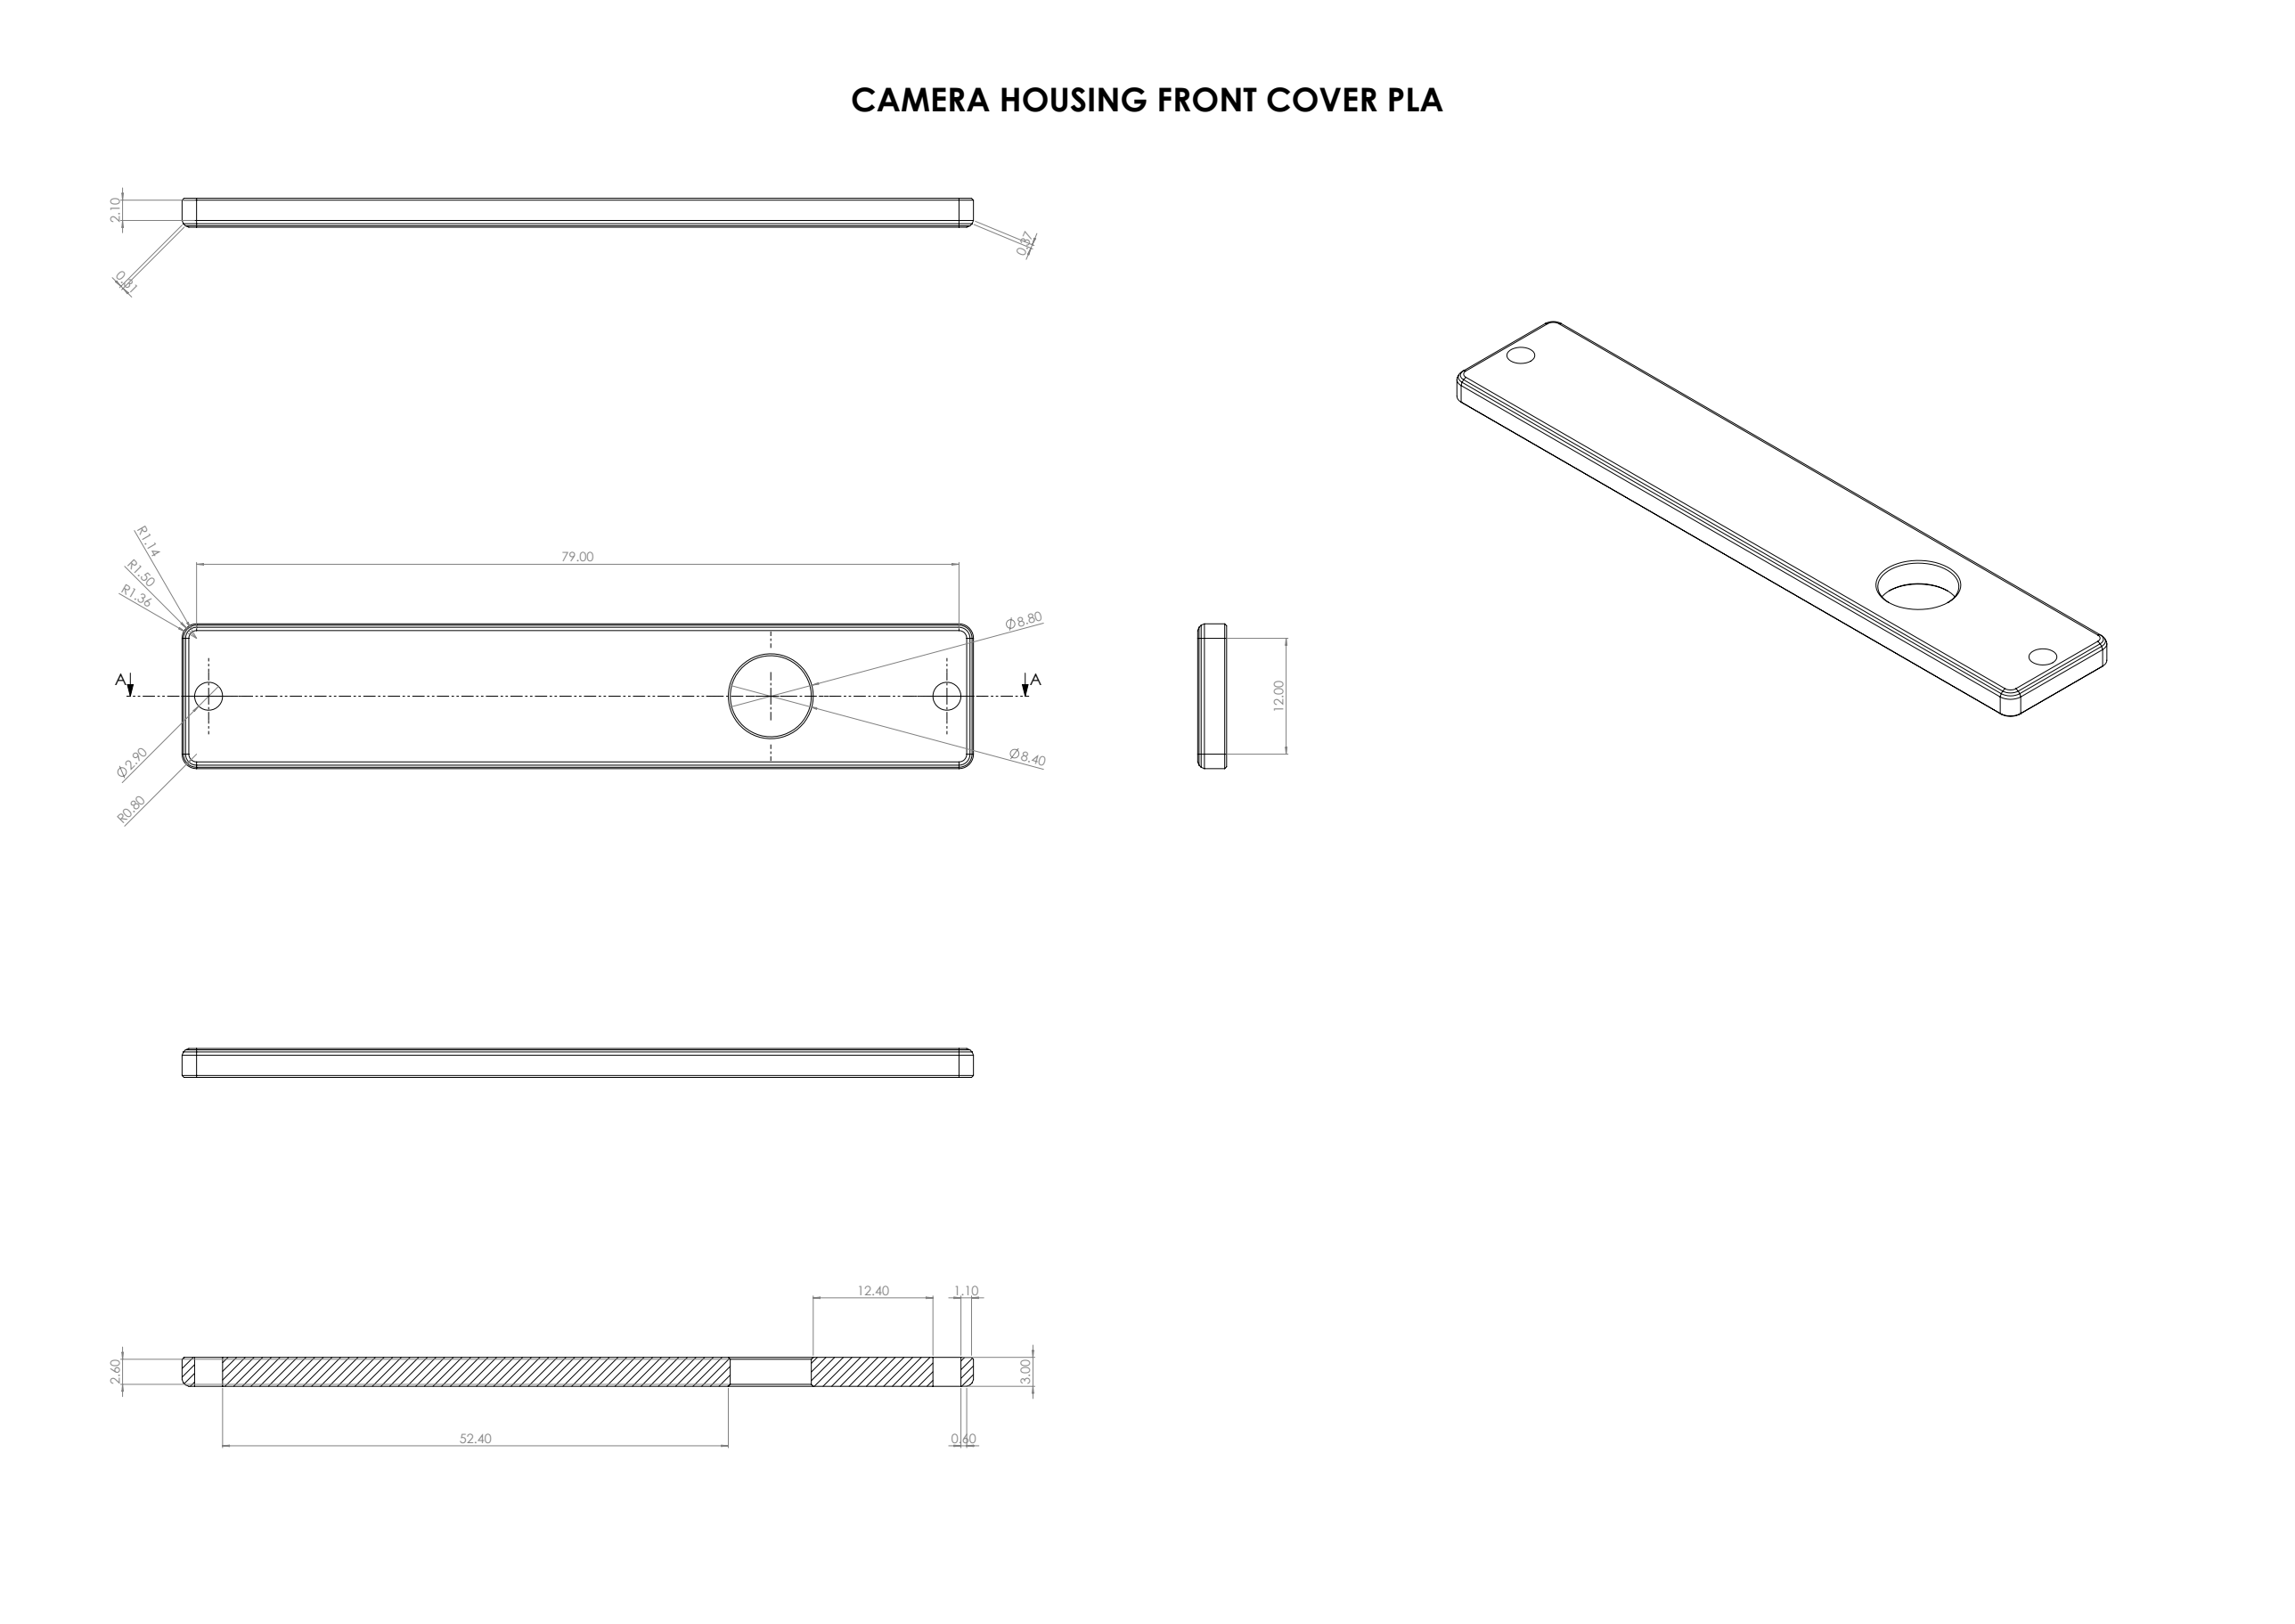
ISO-10303-21;
HEADER;
/* Generated by software containing ST-Developer
 * from STEP Tools, Inc. (www.steptools.com) 
 */

FILE_DESCRIPTION(
/* description */ (''),
/* implementation_level */ '2;1');

FILE_NAME(
/* name */ '04_Camera_Housing_Front_Cover_PLA.step',
/* time_stamp */ '2026-10-21T02:01:14-07:00',
/* author */ (''),
/* organization */ (''),
/* preprocessor_version */ 'ST-DEVELOPER v20.2',
/* originating_system */ 'Autodesk Translation Framework v15.15.0.0',
/* authorisation */ '');

FILE_SCHEMA (('AUTOMOTIVE_DESIGN { 1 0 10303 214 3 1 1 }'));
ENDSEC;

DATA;
#10=MECHANICAL_DESIGN_GEOMETRIC_PRESENTATION_REPRESENTATION('',(#617),#37181);
#591=SHAPE_REPRESENTATION_RELATIONSHIP('SRR','None',#37241,#604);
#604=ADVANCED_BREP_SHAPE_REPRESENTATION('',(#630),#37171);
#617=STYLED_ITEM('',(#37352),#630);
#630=MANIFOLD_SOLID_BREP('Body1',#14779);
#665=FACE_BOUND('',#2517,.T.);
#666=FACE_BOUND('',#2518,.T.);
#667=FACE_BOUND('',#2519,.T.);
#668=FACE_BOUND('',#2522,.T.);
#669=FACE_BOUND('',#2523,.T.);
#670=FACE_BOUND('',#2524,.T.);
#719=CYLINDRICAL_SURFACE('',#15327,4.2);
#720=CYLINDRICAL_SURFACE('',#15357,1.5);
#721=CYLINDRICAL_SURFACE('',#15360,1.5);
#722=CYLINDRICAL_SURFACE('',#15398,1.45);
#723=CYLINDRICAL_SURFACE('',#15399,1.45);
#724=CYLINDRICAL_SURFACE('',#15400,1.5);
#725=CYLINDRICAL_SURFACE('',#15401,1.5);
#1062=CIRCLE('',#15325,4.4);
#1063=CIRCLE('',#15326,4.2);
#1064=CIRCLE('',#15328,4.2);
#1065=CIRCLE('',#15330,1.30000000000001);
#1066=CIRCLE('',#15331,1.30000000000001);
#1067=CIRCLE('',#15332,1.30000000000001);
#1068=CIRCLE('',#15333,1.3);
#1069=CIRCLE('',#15334,1.45);
#1070=CIRCLE('',#15335,1.45);
#1071=CIRCLE('',#15337,4.4);
#1072=CIRCLE('',#15339,0.800000000000008);
#1073=CIRCLE('',#15340,0.800000000000008);
#1074=CIRCLE('',#15341,0.80000000000001);
#1075=CIRCLE('',#15342,0.800000000000012);
#1076=CIRCLE('',#15343,1.45);
#1077=CIRCLE('',#15344,1.45);
#1078=CIRCLE('',#15347,1.5);
#1079=CIRCLE('',#15350,1.5);
#1080=CIRCLE('',#15353,1.5);
#1081=CIRCLE('',#15356,1.5);
#1082=CIRCLE('',#15358,1.5);
#1083=CIRCLE('',#15361,1.5);
#1084=CIRCLE('',#15365,1.35857864376269);
#1085=CIRCLE('',#15368,1.35857864376269);
#1086=CIRCLE('',#15371,1.3585786437627);
#1087=CIRCLE('',#15372,1.5);
#1088=CIRCLE('',#15375,1.35857864376269);
#1089=CIRCLE('',#15376,1.5);
#1090=CIRCLE('',#15378,1.14142135623731);
#1091=CIRCLE('',#15381,1.14142135623731);
#1092=CIRCLE('',#15390,1.1414213562373);
#1093=CIRCLE('',#15393,1.1414213562373);
#1331=CONICAL_SURFACE('',#15324,4.3,0.785398163397448);
#1332=CONICAL_SURFACE('',#15336,4.3,0.785398163397448);
#1333=CONICAL_SURFACE('',#15346,1.4,0.785398163397434);
#1334=CONICAL_SURFACE('',#15349,1.4,0.785398163397434);
#1335=CONICAL_SURFACE('',#15352,1.4,0.785398163397435);
#1336=CONICAL_SURFACE('',#15355,1.4,0.785398163397443);
#1337=CONICAL_SURFACE('',#15364,1.42928932188135,0.392699081698732);
#1338=CONICAL_SURFACE('',#15367,1.42928932188135,0.392699081698732);
#1339=CONICAL_SURFACE('',#15370,1.42928932188135,0.392699081698704);
#1340=CONICAL_SURFACE('',#15374,1.42928932188135,0.392699081698719);
#1341=CONICAL_SURFACE('',#15377,1.25,0.785398163397447);
#1342=CONICAL_SURFACE('',#15380,1.25,0.785398163397444);
#1343=CONICAL_SURFACE('',#15385,0.970710678118663,1.17809724509616);
#1344=CONICAL_SURFACE('',#15387,0.97071067811866,1.17809724509617);
#1345=CONICAL_SURFACE('',#15389,0.970710678118656,1.17809724509617);
#1346=CONICAL_SURFACE('',#15392,0.970710678118656,1.17809724509617);
#1347=CONICAL_SURFACE('',#15394,1.25,0.785398163397447);
#1348=CONICAL_SURFACE('',#15396,1.25,0.785398163397447);
#1649=FACE_OUTER_BOUND('',#2514,.T.);
#1650=FACE_OUTER_BOUND('',#2515,.T.);
#1651=FACE_OUTER_BOUND('',#2516,.T.);
#1652=FACE_OUTER_BOUND('',#2520,.T.);
#1653=FACE_OUTER_BOUND('',#2521,.T.);
#1654=FACE_OUTER_BOUND('',#2525,.T.);
#1655=FACE_OUTER_BOUND('',#2526,.T.);
#1656=FACE_OUTER_BOUND('',#2527,.T.);
#1657=FACE_OUTER_BOUND('',#2528,.T.);
#1658=FACE_OUTER_BOUND('',#2529,.T.);
#1659=FACE_OUTER_BOUND('',#2530,.T.);
#1660=FACE_OUTER_BOUND('',#2531,.T.);
#1661=FACE_OUTER_BOUND('',#2532,.T.);
#1662=FACE_OUTER_BOUND('',#2533,.T.);
#1663=FACE_OUTER_BOUND('',#2534,.T.);
#1664=FACE_OUTER_BOUND('',#2535,.T.);
#1665=FACE_OUTER_BOUND('',#2536,.T.);
#1666=FACE_OUTER_BOUND('',#2537,.T.);
#1667=FACE_OUTER_BOUND('',#2538,.T.);
#1668=FACE_OUTER_BOUND('',#2539,.T.);
#1669=FACE_OUTER_BOUND('',#2540,.T.);
#1670=FACE_OUTER_BOUND('',#2541,.T.);
#1671=FACE_OUTER_BOUND('',#2542,.T.);
#1672=FACE_OUTER_BOUND('',#2543,.T.);
#1673=FACE_OUTER_BOUND('',#2544,.T.);
#1674=FACE_OUTER_BOUND('',#2545,.T.);
#1675=FACE_OUTER_BOUND('',#2546,.T.);
#1676=FACE_OUTER_BOUND('',#2547,.T.);
#1677=FACE_OUTER_BOUND('',#2548,.T.);
#1678=FACE_OUTER_BOUND('',#2549,.T.);
#1679=FACE_OUTER_BOUND('',#2550,.T.);
#1680=FACE_OUTER_BOUND('',#2551,.T.);
#1681=FACE_OUTER_BOUND('',#2552,.T.);
#1682=FACE_OUTER_BOUND('',#2553,.T.);
#1683=FACE_OUTER_BOUND('',#2554,.T.);
#1684=FACE_OUTER_BOUND('',#2555,.T.);
#1685=FACE_OUTER_BOUND('',#2556,.T.);
#1686=FACE_OUTER_BOUND('',#2557,.T.);
#1687=FACE_OUTER_BOUND('',#2558,.T.);
#1688=FACE_OUTER_BOUND('',#2559,.T.);
#1689=FACE_OUTER_BOUND('',#2560,.T.);
#1690=FACE_OUTER_BOUND('',#2561,.T.);
#1691=FACE_OUTER_BOUND('',#2562,.T.);
#1692=FACE_OUTER_BOUND('',#2563,.T.);
#1693=FACE_OUTER_BOUND('',#2564,.T.);
#1694=FACE_OUTER_BOUND('',#2565,.T.);
#1695=FACE_OUTER_BOUND('',#2566,.T.);
#2514=EDGE_LOOP('',(#10539,#10540,#10541,#10542));
#2515=EDGE_LOOP('',(#10543,#10544,#10545,#10546));
#2516=EDGE_LOOP('',(#10547,#10548,#10549,#10550,#10551,#10552,#10553,#10554));
#2517=EDGE_LOOP('',(#10555));
#2518=EDGE_LOOP('',(#10556));
#2519=EDGE_LOOP('',(#10557));
#2520=EDGE_LOOP('',(#10558,#10559,#10560,#10561));
#2521=EDGE_LOOP('',(#10562,#10563,#10564,#10565,#10566,#10567,#10568,#10569));
#2522=EDGE_LOOP('',(#10570));
#2523=EDGE_LOOP('',(#10571));
#2524=EDGE_LOOP('',(#10572));
#2525=EDGE_LOOP('',(#10573,#10574,#10575,#10576));
#2526=EDGE_LOOP('',(#10577,#10578,#10579,#10580));
#2527=EDGE_LOOP('',(#10581,#10582,#10583,#10584));
#2528=EDGE_LOOP('',(#10585,#10586,#10587,#10588));
#2529=EDGE_LOOP('',(#10589,#10590,#10591,#10592));
#2530=EDGE_LOOP('',(#10593,#10594,#10595,#10596));
#2531=EDGE_LOOP('',(#10597,#10598,#10599,#10600));
#2532=EDGE_LOOP('',(#10601,#10602,#10603,#10604));
#2533=EDGE_LOOP('',(#10605,#10606,#10607,#10608));
#2534=EDGE_LOOP('',(#10609,#10610,#10611,#10612));
#2535=EDGE_LOOP('',(#10613,#10614,#10615,#10616));
#2536=EDGE_LOOP('',(#10617,#10618,#10619,#10620));
#2537=EDGE_LOOP('',(#10621,#10622,#10623,#10624));
#2538=EDGE_LOOP('',(#10625,#10626,#10627,#10628));
#2539=EDGE_LOOP('',(#10629,#10630,#10631,#10632));
#2540=EDGE_LOOP('',(#10633,#10634,#10635,#10636));
#2541=EDGE_LOOP('',(#10637,#10638,#10639,#10640));
#2542=EDGE_LOOP('',(#10641,#10642,#10643,#10644));
#2543=EDGE_LOOP('',(#10645,#10646,#10647,#10648));
#2544=EDGE_LOOP('',(#10649,#10650,#10651,#10652));
#2545=EDGE_LOOP('',(#10653,#10654,#10655,#10656));
#2546=EDGE_LOOP('',(#10657,#10658,#10659,#10660));
#2547=EDGE_LOOP('',(#10661,#10662,#10663,#10664));
#2548=EDGE_LOOP('',(#10665,#10666,#10667,#10668));
#2549=EDGE_LOOP('',(#10669,#10670,#10671,#10672));
#2550=EDGE_LOOP('',(#10673,#10674,#10675,#10676));
#2551=EDGE_LOOP('',(#10677,#10678,#10679,#10680));
#2552=EDGE_LOOP('',(#10681,#10682,#10683,#10684));
#2553=EDGE_LOOP('',(#10685,#10686,#10687,#10688));
#2554=EDGE_LOOP('',(#10689,#10690,#10691,#10692));
#2555=EDGE_LOOP('',(#10693,#10694,#10695,#10696));
#2556=EDGE_LOOP('',(#10697,#10698,#10699,#10700));
#2557=EDGE_LOOP('',(#10701,#10702,#10703,#10704));
#2558=EDGE_LOOP('',(#10705,#10706,#10707,#10708));
#2559=EDGE_LOOP('',(#10709,#10710,#10711,#10712));
#2560=EDGE_LOOP('',(#10713,#10714,#10715,#10716));
#2561=EDGE_LOOP('',(#10717,#10718,#10719,#10720));
#2562=EDGE_LOOP('',(#10721,#10722,#10723,#10724));
#2563=EDGE_LOOP('',(#10725,#10726,#10727,#10728));
#2564=EDGE_LOOP('',(#10729,#10730,#10731,#10732));
#2565=EDGE_LOOP('',(#10733,#10734,#10735,#10736));
#2566=EDGE_LOOP('',(#10737,#10738,#10739,#10740));
#3715=LINE('',#21391,#4954);
#3716=LINE('',#21396,#4955);
#3717=LINE('',#21400,#4956);
#3718=LINE('',#21404,#4957);
#3719=LINE('',#21408,#4958);
#3720=LINE('',#21412,#4959);
#3721=LINE('',#21421,#4960);
#3722=LINE('',#21425,#4961);
#3723=LINE('',#21429,#4962);
#3724=LINE('',#21433,#4963);
#3725=LINE('',#21437,#4964);
#3726=LINE('',#21445,#4965);
#3727=LINE('',#21447,#4966);
#3728=LINE('',#21448,#4967);
#3729=LINE('',#21452,#4968);
#3730=LINE('',#21455,#4969);
#3731=LINE('',#21456,#4970);
#3732=LINE('',#21460,#4971);
#3733=LINE('',#21463,#4972);
#3734=LINE('',#21464,#4973);
#3735=LINE('',#21468,#4974);
#3736=LINE('',#21471,#4975);
#3737=LINE('',#21472,#4976);
#3738=LINE('',#21477,#4977);
#3739=LINE('',#21480,#4978);
#3740=LINE('',#21483,#4979);
#3741=LINE('',#21484,#4980);
#3742=LINE('',#21487,#4981);
#3743=LINE('',#21491,#4982);
#3744=LINE('',#21492,#4983);
#3745=LINE('',#21495,#4984);
#3746=LINE('',#21497,#4985);
#3747=LINE('',#21499,#4986);
#3748=LINE('',#21500,#4987);
#3749=LINE('',#21503,#4988);
#3750=LINE('',#21507,#4989);
#3751=LINE('',#21508,#4990);
#3752=LINE('',#21511,#4991);
#3753=LINE('',#21515,#4992);
#3754=LINE('',#21516,#4993);
#3755=LINE('',#21520,#4994);
#3756=LINE('',#21526,#4995);
#3757=LINE('',#21527,#4996);
#3758=LINE('',#21528,#4997);
#3759=LINE('',#21534,#4998);
#3760=LINE('',#21537,#4999);
#3761=LINE('',#21540,#5000);
#3762=LINE('',#21541,#5001);
#3763=LINE('',#21544,#5002);
#3764=LINE('',#21548,#5003);
#3765=LINE('',#21549,#5004);
#3766=LINE('',#21551,#5005);
#3767=LINE('',#21553,#5006);
#3768=LINE('',#21554,#5007);
#3769=LINE('',#21556,#5008);
#3770=LINE('',#21558,#5009);
#3771=LINE('',#21560,#5010);
#3772=LINE('',#21563,#5011);
#3773=LINE('',#21564,#5012);
#3774=LINE('',#21567,#5013);
#3775=LINE('',#21571,#5014);
#3776=LINE('',#21572,#5015);
#3777=LINE('',#21576,#5016);
#3778=LINE('',#21577,#5017);
#3779=LINE('',#21579,#5018);
#3780=LINE('',#21583,#5019);
#3781=LINE('',#21585,#5020);
#3782=LINE('',#21587,#5021);
#3783=LINE('',#21589,#5022);
#4954=VECTOR('',#17423,4.3);
#4955=VECTOR('',#17430,4.2);
#4956=VECTOR('',#17433,10.);
#4957=VECTOR('',#17436,10.);
#4958=VECTOR('',#17439,10.);
#4959=VECTOR('',#17442,10.);
#4960=VECTOR('',#17453,4.3);
#4961=VECTOR('',#17456,10.);
#4962=VECTOR('',#17459,10.);
#4963=VECTOR('',#17462,10.);
#4964=VECTOR('',#17465,10.);
#4965=VECTOR('',#17474,10.);
#4966=VECTOR('',#17475,10.);
#4967=VECTOR('',#17476,10.);
#4968=VECTOR('',#17481,10.);
#4969=VECTOR('',#17484,10.);
#4970=VECTOR('',#17485,10.);
#4971=VECTOR('',#17490,10.);
#4972=VECTOR('',#17493,10.);
#4973=VECTOR('',#17494,10.);
#4974=VECTOR('',#17499,10.);
#4975=VECTOR('',#17502,10.);
#4976=VECTOR('',#17503,10.);
#4977=VECTOR('',#17510,10.);
#4978=VECTOR('',#17513,10.);
#4979=VECTOR('',#17516,10.);
#4980=VECTOR('',#17517,10.);
#4981=VECTOR('',#17520,10.);
#4982=VECTOR('',#17525,10.);
#4983=VECTOR('',#17526,10.);
#4984=VECTOR('',#17529,10.);
#4985=VECTOR('',#17530,10.);
#4986=VECTOR('',#17531,10.);
#4987=VECTOR('',#17532,10.);
#4988=VECTOR('',#17535,10.);
#4989=VECTOR('',#17540,10.);
#4990=VECTOR('',#17541,10.);
#4991=VECTOR('',#17544,10.);
#4992=VECTOR('',#17549,10.);
#4993=VECTOR('',#17550,10.);
#4994=VECTOR('',#17553,10.);
#4995=VECTOR('',#17560,10.);
#4996=VECTOR('',#17561,10.);
#4997=VECTOR('',#17562,10.);
#4998=VECTOR('',#17571,10.);
#4999=VECTOR('',#17574,10.);
#5000=VECTOR('',#17577,10.);
#5001=VECTOR('',#17578,10.);
#5002=VECTOR('',#17581,10.);
#5003=VECTOR('',#17586,10.);
#5004=VECTOR('',#17587,10.);
#5005=VECTOR('',#17590,10.);
#5006=VECTOR('',#17593,10.);
#5007=VECTOR('',#17594,10.);
#5008=VECTOR('',#17597,10.);
#5009=VECTOR('',#17600,10.);
#5010=VECTOR('',#17603,10.);
#5011=VECTOR('',#17606,10.);
#5012=VECTOR('',#17607,10.);
#5013=VECTOR('',#17610,10.);
#5014=VECTOR('',#17615,10.);
#5015=VECTOR('',#17616,10.);
#5016=VECTOR('',#17623,10.);
#5017=VECTOR('',#17624,10.);
#5018=VECTOR('',#17627,10.);
#5019=VECTOR('',#17634,1.45);
#5020=VECTOR('',#17637,1.45);
#5021=VECTOR('',#17640,10.);
#5022=VECTOR('',#17643,10.);
#6095=VERTEX_POINT('',#21388);
#6096=VERTEX_POINT('',#21390);
#6097=VERTEX_POINT('',#21394);
#6098=VERTEX_POINT('',#21398);
#6099=VERTEX_POINT('',#21399);
#6100=VERTEX_POINT('',#21401);
#6101=VERTEX_POINT('',#21403);
#6102=VERTEX_POINT('',#21405);
#6103=VERTEX_POINT('',#21407);
#6104=VERTEX_POINT('',#21409);
#6105=VERTEX_POINT('',#21411);
#6106=VERTEX_POINT('',#21414);
#6107=VERTEX_POINT('',#21416);
#6108=VERTEX_POINT('',#21419);
#6109=VERTEX_POINT('',#21423);
#6110=VERTEX_POINT('',#21424);
#6111=VERTEX_POINT('',#21426);
#6112=VERTEX_POINT('',#21428);
#6113=VERTEX_POINT('',#21430);
#6114=VERTEX_POINT('',#21432);
#6115=VERTEX_POINT('',#21434);
#6116=VERTEX_POINT('',#21436);
#6117=VERTEX_POINT('',#21439);
#6118=VERTEX_POINT('',#21441);
#6119=VERTEX_POINT('',#21444);
#6120=VERTEX_POINT('',#21446);
#6121=VERTEX_POINT('',#21450);
#6122=VERTEX_POINT('',#21454);
#6123=VERTEX_POINT('',#21458);
#6124=VERTEX_POINT('',#21462);
#6125=VERTEX_POINT('',#21466);
#6126=VERTEX_POINT('',#21470);
#6127=VERTEX_POINT('',#21476);
#6128=VERTEX_POINT('',#21478);
#6129=VERTEX_POINT('',#21482);
#6130=VERTEX_POINT('',#21486);
#6131=VERTEX_POINT('',#21490);
#6132=VERTEX_POINT('',#21494);
#6133=VERTEX_POINT('',#21496);
#6134=VERTEX_POINT('',#21498);
#6135=VERTEX_POINT('',#21502);
#6136=VERTEX_POINT('',#21506);
#6137=VERTEX_POINT('',#21510);
#6138=VERTEX_POINT('',#21514);
#6139=VERTEX_POINT('',#21518);
#6140=VERTEX_POINT('',#21519);
#6141=VERTEX_POINT('',#21524);
#6142=VERTEX_POINT('',#21525);
#6143=VERTEX_POINT('',#21533);
#6144=VERTEX_POINT('',#21535);
#6145=VERTEX_POINT('',#21539);
#6146=VERTEX_POINT('',#21543);
#6147=VERTEX_POINT('',#21547);
#6148=VERTEX_POINT('',#21562);
#6149=VERTEX_POINT('',#21566);
#6150=VERTEX_POINT('',#21570);
#7711=EDGE_CURVE('',#6095,#6095,#1062,.T.);
#7712=EDGE_CURVE('',#6095,#6096,#3715,.T.);
#7713=EDGE_CURVE('',#6096,#6096,#1063,.T.);
#7714=EDGE_CURVE('',#6097,#6097,#1064,.T.);
#7715=EDGE_CURVE('',#6097,#6096,#3716,.T.);
#7716=EDGE_CURVE('',#6098,#6099,#3717,.T.);
#7717=EDGE_CURVE('',#6100,#6098,#1065,.T.);
#7718=EDGE_CURVE('',#6101,#6100,#3718,.T.);
#7719=EDGE_CURVE('',#6102,#6101,#1066,.T.);
#7720=EDGE_CURVE('',#6103,#6102,#3719,.T.);
#7721=EDGE_CURVE('',#6104,#6103,#1067,.T.);
#7722=EDGE_CURVE('',#6105,#6104,#3720,.T.);
#7723=EDGE_CURVE('',#6099,#6105,#1068,.T.);
#7724=EDGE_CURVE('',#6106,#6106,#1069,.T.);
#7725=EDGE_CURVE('',#6107,#6107,#1070,.T.);
#7726=EDGE_CURVE('',#6108,#6108,#1071,.T.);
#7727=EDGE_CURVE('',#6108,#6097,#3721,.T.);
#7728=EDGE_CURVE('',#6109,#6110,#3722,.T.);
#7729=EDGE_CURVE('',#6111,#6109,#1072,.T.);
#7730=EDGE_CURVE('',#6112,#6111,#3723,.T.);
#7731=EDGE_CURVE('',#6113,#6112,#1073,.T.);
#7732=EDGE_CURVE('',#6114,#6113,#3724,.T.);
#7733=EDGE_CURVE('',#6115,#6114,#1074,.T.);
#7734=EDGE_CURVE('',#6116,#6115,#3725,.T.);
#7735=EDGE_CURVE('',#6110,#6116,#1075,.T.);
#7736=EDGE_CURVE('',#6117,#6117,#1076,.T.);
#7737=EDGE_CURVE('',#6118,#6118,#1077,.T.);
#7738=EDGE_CURVE('',#6119,#6098,#3726,.T.);
#7739=EDGE_CURVE('',#6099,#6120,#3727,.T.);
#7740=EDGE_CURVE('',#6120,#6119,#3728,.T.);
#7741=EDGE_CURVE('',#6119,#6121,#1078,.T.);
#7742=EDGE_CURVE('',#6121,#6100,#3729,.T.);
#7743=EDGE_CURVE('',#6122,#6101,#3730,.T.);
#7744=EDGE_CURVE('',#6121,#6122,#3731,.T.);
#7745=EDGE_CURVE('',#6122,#6123,#1079,.T.);
#7746=EDGE_CURVE('',#6123,#6102,#3732,.T.);
#7747=EDGE_CURVE('',#6124,#6103,#3733,.T.);
#7748=EDGE_CURVE('',#6123,#6124,#3734,.T.);
#7749=EDGE_CURVE('',#6124,#6125,#1080,.T.);
#7750=EDGE_CURVE('',#6125,#6104,#3735,.T.);
#7751=EDGE_CURVE('',#6126,#6105,#3736,.T.);
#7752=EDGE_CURVE('',#6125,#6126,#3737,.T.);
#7753=EDGE_CURVE('',#6126,#6120,#1081,.T.);
#7754=EDGE_CURVE('',#6122,#6127,#3738,.T.);
#7755=EDGE_CURVE('',#6128,#6127,#1082,.T.);
#7756=EDGE_CURVE('',#6128,#6123,#3739,.T.);
#7757=EDGE_CURVE('',#6129,#6121,#3740,.T.);
#7758=EDGE_CURVE('',#6127,#6129,#3741,.T.);
#7759=EDGE_CURVE('',#6119,#6130,#3742,.T.);
#7760=EDGE_CURVE('',#6129,#6130,#1083,.T.);
#7761=EDGE_CURVE('',#6131,#6120,#3743,.T.);
#7762=EDGE_CURVE('',#6130,#6131,#3744,.T.);
#7763=EDGE_CURVE('',#6128,#6132,#3745,.T.);
#7764=EDGE_CURVE('',#6132,#6133,#3746,.T.);
#7765=EDGE_CURVE('',#6133,#6134,#3747,.T.);
#7766=EDGE_CURVE('',#6134,#6128,#3748,.T.);
#7767=EDGE_CURVE('',#6127,#6135,#3749,.T.);
#7768=EDGE_CURVE('',#6135,#6132,#1084,.T.);
#7769=EDGE_CURVE('',#6129,#6136,#3750,.T.);
#7770=EDGE_CURVE('',#6136,#6135,#3751,.T.);
#7771=EDGE_CURVE('',#6130,#6137,#3752,.T.);
#7772=EDGE_CURVE('',#6137,#6136,#1085,.T.);
#7773=EDGE_CURVE('',#6131,#6138,#3753,.T.);
#7774=EDGE_CURVE('',#6138,#6137,#3754,.T.);
#7775=EDGE_CURVE('',#6139,#6140,#3755,.T.);
#7776=EDGE_CURVE('',#6140,#6138,#1086,.T.);
#7777=EDGE_CURVE('',#6131,#6139,#1087,.T.);
#7778=EDGE_CURVE('',#6141,#6142,#3756,.T.);
#7779=EDGE_CURVE('',#6142,#6140,#3757,.T.);
#7780=EDGE_CURVE('',#6139,#6141,#3758,.T.);
#7781=EDGE_CURVE('',#6133,#6142,#1088,.T.);
#7782=EDGE_CURVE('',#6141,#6134,#1089,.T.);
#7783=EDGE_CURVE('',#6143,#6140,#3759,.T.);
#7784=EDGE_CURVE('',#6144,#6143,#1090,.T.);
#7785=EDGE_CURVE('',#6144,#6138,#3760,.T.);
#7786=EDGE_CURVE('',#6145,#6142,#3761,.T.);
#7787=EDGE_CURVE('',#6143,#6145,#3762,.T.);
#7788=EDGE_CURVE('',#6146,#6133,#3763,.T.);
#7789=EDGE_CURVE('',#6145,#6146,#1091,.T.);
#7790=EDGE_CURVE('',#6147,#6132,#3764,.T.);
#7791=EDGE_CURVE('',#6146,#6147,#3765,.T.);
#7792=EDGE_CURVE('',#6124,#6134,#3766,.T.);
#7793=EDGE_CURVE('',#6110,#6146,#3767,.T.);
#7794=EDGE_CURVE('',#6147,#6109,#3768,.T.);
#7795=EDGE_CURVE('',#6116,#6145,#3769,.T.);
#7796=EDGE_CURVE('',#6115,#6143,#3770,.T.);
#7797=EDGE_CURVE('',#6114,#6144,#3771,.T.);
#7798=EDGE_CURVE('',#6113,#6148,#3772,.T.);
#7799=EDGE_CURVE('',#6148,#6144,#3773,.T.);
#7800=EDGE_CURVE('',#6112,#6149,#3774,.T.);
#7801=EDGE_CURVE('',#6149,#6148,#1092,.T.);
#7802=EDGE_CURVE('',#6111,#6150,#3775,.T.);
#7803=EDGE_CURVE('',#6150,#6149,#3776,.T.);
#7804=EDGE_CURVE('',#6147,#6150,#1093,.T.);
#7805=EDGE_CURVE('',#6148,#6137,#3777,.T.);
#7806=EDGE_CURVE('',#6149,#6136,#3778,.T.);
#7807=EDGE_CURVE('',#6135,#6150,#3779,.T.);
#7808=EDGE_CURVE('',#6118,#6106,#3780,.T.);
#7809=EDGE_CURVE('',#6117,#6107,#3781,.T.);
#7810=EDGE_CURVE('',#6126,#6139,#3782,.T.);
#7811=EDGE_CURVE('',#6141,#6125,#3783,.T.);
#10539=ORIENTED_EDGE('',*,*,#7711,.T.);
#10540=ORIENTED_EDGE('',*,*,#7712,.T.);
#10541=ORIENTED_EDGE('',*,*,#7713,.T.);
#10542=ORIENTED_EDGE('',*,*,#7712,.F.);
#10543=ORIENTED_EDGE('',*,*,#7714,.F.);
#10544=ORIENTED_EDGE('',*,*,#7715,.T.);
#10545=ORIENTED_EDGE('',*,*,#7713,.F.);
#10546=ORIENTED_EDGE('',*,*,#7715,.F.);
#10547=ORIENTED_EDGE('',*,*,#7716,.F.);
#10548=ORIENTED_EDGE('',*,*,#7717,.F.);
#10549=ORIENTED_EDGE('',*,*,#7718,.F.);
#10550=ORIENTED_EDGE('',*,*,#7719,.F.);
#10551=ORIENTED_EDGE('',*,*,#7720,.F.);
#10552=ORIENTED_EDGE('',*,*,#7721,.F.);
#10553=ORIENTED_EDGE('',*,*,#7722,.F.);
#10554=ORIENTED_EDGE('',*,*,#7723,.F.);
#10555=ORIENTED_EDGE('',*,*,#7724,.T.);
#10556=ORIENTED_EDGE('',*,*,#7725,.T.);
#10557=ORIENTED_EDGE('',*,*,#7711,.F.);
#10558=ORIENTED_EDGE('',*,*,#7726,.T.);
#10559=ORIENTED_EDGE('',*,*,#7727,.T.);
#10560=ORIENTED_EDGE('',*,*,#7714,.T.);
#10561=ORIENTED_EDGE('',*,*,#7727,.F.);
#10562=ORIENTED_EDGE('',*,*,#7728,.F.);
#10563=ORIENTED_EDGE('',*,*,#7729,.F.);
#10564=ORIENTED_EDGE('',*,*,#7730,.F.);
#10565=ORIENTED_EDGE('',*,*,#7731,.F.);
#10566=ORIENTED_EDGE('',*,*,#7732,.F.);
#10567=ORIENTED_EDGE('',*,*,#7733,.F.);
#10568=ORIENTED_EDGE('',*,*,#7734,.F.);
#10569=ORIENTED_EDGE('',*,*,#7735,.F.);
#10570=ORIENTED_EDGE('',*,*,#7736,.T.);
#10571=ORIENTED_EDGE('',*,*,#7737,.T.);
#10572=ORIENTED_EDGE('',*,*,#7726,.F.);
#10573=ORIENTED_EDGE('',*,*,#7738,.T.);
#10574=ORIENTED_EDGE('',*,*,#7716,.T.);
#10575=ORIENTED_EDGE('',*,*,#7739,.T.);
#10576=ORIENTED_EDGE('',*,*,#7740,.T.);
#10577=ORIENTED_EDGE('',*,*,#7738,.F.);
#10578=ORIENTED_EDGE('',*,*,#7741,.T.);
#10579=ORIENTED_EDGE('',*,*,#7742,.T.);
#10580=ORIENTED_EDGE('',*,*,#7717,.T.);
#10581=ORIENTED_EDGE('',*,*,#7743,.T.);
#10582=ORIENTED_EDGE('',*,*,#7718,.T.);
#10583=ORIENTED_EDGE('',*,*,#7742,.F.);
#10584=ORIENTED_EDGE('',*,*,#7744,.T.);
#10585=ORIENTED_EDGE('',*,*,#7743,.F.);
#10586=ORIENTED_EDGE('',*,*,#7745,.T.);
#10587=ORIENTED_EDGE('',*,*,#7746,.T.);
#10588=ORIENTED_EDGE('',*,*,#7719,.T.);
#10589=ORIENTED_EDGE('',*,*,#7747,.T.);
#10590=ORIENTED_EDGE('',*,*,#7720,.T.);
#10591=ORIENTED_EDGE('',*,*,#7746,.F.);
#10592=ORIENTED_EDGE('',*,*,#7748,.T.);
#10593=ORIENTED_EDGE('',*,*,#7747,.F.);
#10594=ORIENTED_EDGE('',*,*,#7749,.T.);
#10595=ORIENTED_EDGE('',*,*,#7750,.T.);
#10596=ORIENTED_EDGE('',*,*,#7721,.T.);
#10597=ORIENTED_EDGE('',*,*,#7751,.T.);
#10598=ORIENTED_EDGE('',*,*,#7722,.T.);
#10599=ORIENTED_EDGE('',*,*,#7750,.F.);
#10600=ORIENTED_EDGE('',*,*,#7752,.T.);
#10601=ORIENTED_EDGE('',*,*,#7751,.F.);
#10602=ORIENTED_EDGE('',*,*,#7753,.T.);
#10603=ORIENTED_EDGE('',*,*,#7739,.F.);
#10604=ORIENTED_EDGE('',*,*,#7723,.T.);
#10605=ORIENTED_EDGE('',*,*,#7745,.F.);
#10606=ORIENTED_EDGE('',*,*,#7754,.T.);
#10607=ORIENTED_EDGE('',*,*,#7755,.F.);
#10608=ORIENTED_EDGE('',*,*,#7756,.T.);
#10609=ORIENTED_EDGE('',*,*,#7744,.F.);
#10610=ORIENTED_EDGE('',*,*,#7757,.F.);
#10611=ORIENTED_EDGE('',*,*,#7758,.F.);
#10612=ORIENTED_EDGE('',*,*,#7754,.F.);
#10613=ORIENTED_EDGE('',*,*,#7741,.F.);
#10614=ORIENTED_EDGE('',*,*,#7759,.T.);
#10615=ORIENTED_EDGE('',*,*,#7760,.F.);
#10616=ORIENTED_EDGE('',*,*,#7757,.T.);
#10617=ORIENTED_EDGE('',*,*,#7740,.F.);
#10618=ORIENTED_EDGE('',*,*,#7761,.F.);
#10619=ORIENTED_EDGE('',*,*,#7762,.F.);
#10620=ORIENTED_EDGE('',*,*,#7759,.F.);
#10621=ORIENTED_EDGE('',*,*,#7763,.T.);
#10622=ORIENTED_EDGE('',*,*,#7764,.T.);
#10623=ORIENTED_EDGE('',*,*,#7765,.T.);
#10624=ORIENTED_EDGE('',*,*,#7766,.T.);
#10625=ORIENTED_EDGE('',*,*,#7767,.T.);
#10626=ORIENTED_EDGE('',*,*,#7768,.T.);
#10627=ORIENTED_EDGE('',*,*,#7763,.F.);
#10628=ORIENTED_EDGE('',*,*,#7755,.T.);
#10629=ORIENTED_EDGE('',*,*,#7769,.T.);
#10630=ORIENTED_EDGE('',*,*,#7770,.T.);
#10631=ORIENTED_EDGE('',*,*,#7767,.F.);
#10632=ORIENTED_EDGE('',*,*,#7758,.T.);
#10633=ORIENTED_EDGE('',*,*,#7771,.T.);
#10634=ORIENTED_EDGE('',*,*,#7772,.T.);
#10635=ORIENTED_EDGE('',*,*,#7769,.F.);
#10636=ORIENTED_EDGE('',*,*,#7760,.T.);
#10637=ORIENTED_EDGE('',*,*,#7773,.T.);
#10638=ORIENTED_EDGE('',*,*,#7774,.T.);
#10639=ORIENTED_EDGE('',*,*,#7771,.F.);
#10640=ORIENTED_EDGE('',*,*,#7762,.T.);
#10641=ORIENTED_EDGE('',*,*,#7775,.T.);
#10642=ORIENTED_EDGE('',*,*,#7776,.T.);
#10643=ORIENTED_EDGE('',*,*,#7773,.F.);
#10644=ORIENTED_EDGE('',*,*,#7777,.T.);
#10645=ORIENTED_EDGE('',*,*,#7778,.T.);
#10646=ORIENTED_EDGE('',*,*,#7779,.T.);
#10647=ORIENTED_EDGE('',*,*,#7775,.F.);
#10648=ORIENTED_EDGE('',*,*,#7780,.T.);
#10649=ORIENTED_EDGE('',*,*,#7765,.F.);
#10650=ORIENTED_EDGE('',*,*,#7781,.T.);
#10651=ORIENTED_EDGE('',*,*,#7778,.F.);
#10652=ORIENTED_EDGE('',*,*,#7782,.T.);
#10653=ORIENTED_EDGE('',*,*,#7776,.F.);
#10654=ORIENTED_EDGE('',*,*,#7783,.F.);
#10655=ORIENTED_EDGE('',*,*,#7784,.F.);
#10656=ORIENTED_EDGE('',*,*,#7785,.T.);
#10657=ORIENTED_EDGE('',*,*,#7779,.F.);
#10658=ORIENTED_EDGE('',*,*,#7786,.F.);
#10659=ORIENTED_EDGE('',*,*,#7787,.F.);
#10660=ORIENTED_EDGE('',*,*,#7783,.T.);
#10661=ORIENTED_EDGE('',*,*,#7781,.F.);
#10662=ORIENTED_EDGE('',*,*,#7788,.F.);
#10663=ORIENTED_EDGE('',*,*,#7789,.F.);
#10664=ORIENTED_EDGE('',*,*,#7786,.T.);
#10665=ORIENTED_EDGE('',*,*,#7764,.F.);
#10666=ORIENTED_EDGE('',*,*,#7790,.F.);
#10667=ORIENTED_EDGE('',*,*,#7791,.F.);
#10668=ORIENTED_EDGE('',*,*,#7788,.T.);
#10669=ORIENTED_EDGE('',*,*,#7748,.F.);
#10670=ORIENTED_EDGE('',*,*,#7756,.F.);
#10671=ORIENTED_EDGE('',*,*,#7766,.F.);
#10672=ORIENTED_EDGE('',*,*,#7792,.F.);
#10673=ORIENTED_EDGE('',*,*,#7793,.T.);
#10674=ORIENTED_EDGE('',*,*,#7791,.T.);
#10675=ORIENTED_EDGE('',*,*,#7794,.T.);
#10676=ORIENTED_EDGE('',*,*,#7728,.T.);
#10677=ORIENTED_EDGE('',*,*,#7795,.T.);
#10678=ORIENTED_EDGE('',*,*,#7789,.T.);
#10679=ORIENTED_EDGE('',*,*,#7793,.F.);
#10680=ORIENTED_EDGE('',*,*,#7735,.T.);
#10681=ORIENTED_EDGE('',*,*,#7796,.T.);
#10682=ORIENTED_EDGE('',*,*,#7787,.T.);
#10683=ORIENTED_EDGE('',*,*,#7795,.F.);
#10684=ORIENTED_EDGE('',*,*,#7734,.T.);
#10685=ORIENTED_EDGE('',*,*,#7797,.T.);
#10686=ORIENTED_EDGE('',*,*,#7784,.T.);
#10687=ORIENTED_EDGE('',*,*,#7796,.F.);
#10688=ORIENTED_EDGE('',*,*,#7733,.T.);
#10689=ORIENTED_EDGE('',*,*,#7798,.T.);
#10690=ORIENTED_EDGE('',*,*,#7799,.T.);
#10691=ORIENTED_EDGE('',*,*,#7797,.F.);
#10692=ORIENTED_EDGE('',*,*,#7732,.T.);
#10693=ORIENTED_EDGE('',*,*,#7800,.T.);
#10694=ORIENTED_EDGE('',*,*,#7801,.T.);
#10695=ORIENTED_EDGE('',*,*,#7798,.F.);
#10696=ORIENTED_EDGE('',*,*,#7731,.T.);
#10697=ORIENTED_EDGE('',*,*,#7802,.T.);
#10698=ORIENTED_EDGE('',*,*,#7803,.T.);
#10699=ORIENTED_EDGE('',*,*,#7800,.F.);
#10700=ORIENTED_EDGE('',*,*,#7730,.T.);
#10701=ORIENTED_EDGE('',*,*,#7794,.F.);
#10702=ORIENTED_EDGE('',*,*,#7804,.T.);
#10703=ORIENTED_EDGE('',*,*,#7802,.F.);
#10704=ORIENTED_EDGE('',*,*,#7729,.T.);
#10705=ORIENTED_EDGE('',*,*,#7772,.F.);
#10706=ORIENTED_EDGE('',*,*,#7805,.F.);
#10707=ORIENTED_EDGE('',*,*,#7801,.F.);
#10708=ORIENTED_EDGE('',*,*,#7806,.T.);
#10709=ORIENTED_EDGE('',*,*,#7770,.F.);
#10710=ORIENTED_EDGE('',*,*,#7806,.F.);
#10711=ORIENTED_EDGE('',*,*,#7803,.F.);
#10712=ORIENTED_EDGE('',*,*,#7807,.F.);
#10713=ORIENTED_EDGE('',*,*,#7768,.F.);
#10714=ORIENTED_EDGE('',*,*,#7807,.T.);
#10715=ORIENTED_EDGE('',*,*,#7804,.F.);
#10716=ORIENTED_EDGE('',*,*,#7790,.T.);
#10717=ORIENTED_EDGE('',*,*,#7774,.F.);
#10718=ORIENTED_EDGE('',*,*,#7785,.F.);
#10719=ORIENTED_EDGE('',*,*,#7799,.F.);
#10720=ORIENTED_EDGE('',*,*,#7805,.T.);
#10721=ORIENTED_EDGE('',*,*,#7737,.F.);
#10722=ORIENTED_EDGE('',*,*,#7808,.T.);
#10723=ORIENTED_EDGE('',*,*,#7724,.F.);
#10724=ORIENTED_EDGE('',*,*,#7808,.F.);
#10725=ORIENTED_EDGE('',*,*,#7736,.F.);
#10726=ORIENTED_EDGE('',*,*,#7809,.T.);
#10727=ORIENTED_EDGE('',*,*,#7725,.F.);
#10728=ORIENTED_EDGE('',*,*,#7809,.F.);
#10729=ORIENTED_EDGE('',*,*,#7753,.F.);
#10730=ORIENTED_EDGE('',*,*,#7810,.T.);
#10731=ORIENTED_EDGE('',*,*,#7777,.F.);
#10732=ORIENTED_EDGE('',*,*,#7761,.T.);
#10733=ORIENTED_EDGE('',*,*,#7749,.F.);
#10734=ORIENTED_EDGE('',*,*,#7792,.T.);
#10735=ORIENTED_EDGE('',*,*,#7782,.F.);
#10736=ORIENTED_EDGE('',*,*,#7811,.T.);
#10737=ORIENTED_EDGE('',*,*,#7752,.F.);
#10738=ORIENTED_EDGE('',*,*,#7811,.F.);
#10739=ORIENTED_EDGE('',*,*,#7780,.F.);
#10740=ORIENTED_EDGE('',*,*,#7810,.F.);
#13657=PLANE('',#15329);
#13658=PLANE('',#15338);
#13659=PLANE('',#15345);
#13660=PLANE('',#15348);
#13661=PLANE('',#15351);
#13662=PLANE('',#15354);
#13663=PLANE('',#15359);
#13664=PLANE('',#15362);
#13665=PLANE('',#15363);
#13666=PLANE('',#15366);
#13667=PLANE('',#15369);
#13668=PLANE('',#15373);
#13669=PLANE('',#15379);
#13670=PLANE('',#15382);
#13671=PLANE('',#15383);
#13672=PLANE('',#15384);
#13673=PLANE('',#15386);
#13674=PLANE('',#15388);
#13675=PLANE('',#15391);
#13676=PLANE('',#15395);
#13677=PLANE('',#15397);
#13678=PLANE('',#15402);
#14217=ADVANCED_FACE('',(#1649),#1331,.F.);
#14218=ADVANCED_FACE('',(#1650),#719,.F.);
#14219=ADVANCED_FACE('',(#1651,#665,#666,#667),#13657,.F.);
#14220=ADVANCED_FACE('',(#1652),#1332,.F.);
#14221=ADVANCED_FACE('',(#1653,#668,#669,#670),#13658,.T.);
#14222=ADVANCED_FACE('',(#1654),#13659,.T.);
#14223=ADVANCED_FACE('',(#1655),#1333,.T.);
#14224=ADVANCED_FACE('',(#1656),#13660,.T.);
#14225=ADVANCED_FACE('',(#1657),#1334,.T.);
#14226=ADVANCED_FACE('',(#1658),#13661,.T.);
#14227=ADVANCED_FACE('',(#1659),#1335,.T.);
#14228=ADVANCED_FACE('',(#1660),#13662,.T.);
#14229=ADVANCED_FACE('',(#1661),#1336,.T.);
#14230=ADVANCED_FACE('',(#1662),#720,.T.);
#14231=ADVANCED_FACE('',(#1663),#13663,.T.);
#14232=ADVANCED_FACE('',(#1664),#721,.T.);
#14233=ADVANCED_FACE('',(#1665),#13664,.T.);
#14234=ADVANCED_FACE('',(#1666),#13665,.T.);
#14235=ADVANCED_FACE('',(#1667),#1337,.T.);
#14236=ADVANCED_FACE('',(#1668),#13666,.T.);
#14237=ADVANCED_FACE('',(#1669),#1338,.T.);
#14238=ADVANCED_FACE('',(#1670),#13667,.T.);
#14239=ADVANCED_FACE('',(#1671),#1339,.T.);
#14240=ADVANCED_FACE('',(#1672),#13668,.T.);
#14241=ADVANCED_FACE('',(#1673),#1340,.T.);
#14242=ADVANCED_FACE('',(#1674),#1341,.T.);
#14243=ADVANCED_FACE('',(#1675),#13669,.T.);
#14244=ADVANCED_FACE('',(#1676),#1342,.T.);
#14245=ADVANCED_FACE('',(#1677),#13670,.T.);
#14246=ADVANCED_FACE('',(#1678),#13671,.T.);
#14247=ADVANCED_FACE('',(#1679),#13672,.T.);
#14248=ADVANCED_FACE('',(#1680),#1343,.T.);
#14249=ADVANCED_FACE('',(#1681),#13673,.T.);
#14250=ADVANCED_FACE('',(#1682),#1344,.T.);
#14251=ADVANCED_FACE('',(#1683),#13674,.T.);
#14252=ADVANCED_FACE('',(#1684),#1345,.T.);
#14253=ADVANCED_FACE('',(#1685),#13675,.T.);
#14254=ADVANCED_FACE('',(#1686),#1346,.T.);
#14255=ADVANCED_FACE('',(#1687),#1347,.T.);
#14256=ADVANCED_FACE('',(#1688),#13676,.T.);
#14257=ADVANCED_FACE('',(#1689),#1348,.T.);
#14258=ADVANCED_FACE('',(#1690),#13677,.T.);
#14259=ADVANCED_FACE('',(#1691),#722,.F.);
#14260=ADVANCED_FACE('',(#1692),#723,.F.);
#14261=ADVANCED_FACE('',(#1693),#724,.T.);
#14262=ADVANCED_FACE('',(#1694),#725,.T.);
#14263=ADVANCED_FACE('',(#1695),#13678,.T.);
#14779=CLOSED_SHELL('',(#14217,#14218,#14219,#14220,#14221,#14222,#14223,
#14224,#14225,#14226,#14227,#14228,#14229,#14230,#14231,#14232,#14233,#14234,
#14235,#14236,#14237,#14238,#14239,#14240,#14241,#14242,#14243,#14244,#14245,
#14246,#14247,#14248,#14249,#14250,#14251,#14252,#14253,#14254,#14255,#14256,
#14257,#14258,#14259,#14260,#14261,#14262,#14263));
#15323=AXIS2_PLACEMENT_3D('',#21386,#17417,#17418);
#15324=AXIS2_PLACEMENT_3D('',#21387,#17419,#17420);
#15325=AXIS2_PLACEMENT_3D('',#21389,#17421,#17422);
#15326=AXIS2_PLACEMENT_3D('',#21392,#17424,#17425);
#15327=AXIS2_PLACEMENT_3D('',#21393,#17426,#17427);
#15328=AXIS2_PLACEMENT_3D('',#21395,#17428,#17429);
#15329=AXIS2_PLACEMENT_3D('',#21397,#17431,#17432);
#15330=AXIS2_PLACEMENT_3D('',#21402,#17434,#17435);
#15331=AXIS2_PLACEMENT_3D('',#21406,#17437,#17438);
#15332=AXIS2_PLACEMENT_3D('',#21410,#17440,#17441);
#15333=AXIS2_PLACEMENT_3D('',#21413,#17443,#17444);
#15334=AXIS2_PLACEMENT_3D('',#21415,#17445,#17446);
#15335=AXIS2_PLACEMENT_3D('',#21417,#17447,#17448);
#15336=AXIS2_PLACEMENT_3D('',#21418,#17449,#17450);
#15337=AXIS2_PLACEMENT_3D('',#21420,#17451,#17452);
#15338=AXIS2_PLACEMENT_3D('',#21422,#17454,#17455);
#15339=AXIS2_PLACEMENT_3D('',#21427,#17457,#17458);
#15340=AXIS2_PLACEMENT_3D('',#21431,#17460,#17461);
#15341=AXIS2_PLACEMENT_3D('',#21435,#17463,#17464);
#15342=AXIS2_PLACEMENT_3D('',#21438,#17466,#17467);
#15343=AXIS2_PLACEMENT_3D('',#21440,#17468,#17469);
#15344=AXIS2_PLACEMENT_3D('',#21442,#17470,#17471);
#15345=AXIS2_PLACEMENT_3D('',#21443,#17472,#17473);
#15346=AXIS2_PLACEMENT_3D('',#21449,#17477,#17478);
#15347=AXIS2_PLACEMENT_3D('',#21451,#17479,#17480);
#15348=AXIS2_PLACEMENT_3D('',#21453,#17482,#17483);
#15349=AXIS2_PLACEMENT_3D('',#21457,#17486,#17487);
#15350=AXIS2_PLACEMENT_3D('',#21459,#17488,#17489);
#15351=AXIS2_PLACEMENT_3D('',#21461,#17491,#17492);
#15352=AXIS2_PLACEMENT_3D('',#21465,#17495,#17496);
#15353=AXIS2_PLACEMENT_3D('',#21467,#17497,#17498);
#15354=AXIS2_PLACEMENT_3D('',#21469,#17500,#17501);
#15355=AXIS2_PLACEMENT_3D('',#21473,#17504,#17505);
#15356=AXIS2_PLACEMENT_3D('',#21474,#17506,#17507);
#15357=AXIS2_PLACEMENT_3D('',#21475,#17508,#17509);
#15358=AXIS2_PLACEMENT_3D('',#21479,#17511,#17512);
#15359=AXIS2_PLACEMENT_3D('',#21481,#17514,#17515);
#15360=AXIS2_PLACEMENT_3D('',#21485,#17518,#17519);
#15361=AXIS2_PLACEMENT_3D('',#21488,#17521,#17522);
#15362=AXIS2_PLACEMENT_3D('',#21489,#17523,#17524);
#15363=AXIS2_PLACEMENT_3D('',#21493,#17527,#17528);
#15364=AXIS2_PLACEMENT_3D('',#21501,#17533,#17534);
#15365=AXIS2_PLACEMENT_3D('',#21504,#17536,#17537);
#15366=AXIS2_PLACEMENT_3D('',#21505,#17538,#17539);
#15367=AXIS2_PLACEMENT_3D('',#21509,#17542,#17543);
#15368=AXIS2_PLACEMENT_3D('',#21512,#17545,#17546);
#15369=AXIS2_PLACEMENT_3D('',#21513,#17547,#17548);
#15370=AXIS2_PLACEMENT_3D('',#21517,#17551,#17552);
#15371=AXIS2_PLACEMENT_3D('',#21521,#17554,#17555);
#15372=AXIS2_PLACEMENT_3D('',#21522,#17556,#17557);
#15373=AXIS2_PLACEMENT_3D('',#21523,#17558,#17559);
#15374=AXIS2_PLACEMENT_3D('',#21529,#17563,#17564);
#15375=AXIS2_PLACEMENT_3D('',#21530,#17565,#17566);
#15376=AXIS2_PLACEMENT_3D('',#21531,#17567,#17568);
#15377=AXIS2_PLACEMENT_3D('',#21532,#17569,#17570);
#15378=AXIS2_PLACEMENT_3D('',#21536,#17572,#17573);
#15379=AXIS2_PLACEMENT_3D('',#21538,#17575,#17576);
#15380=AXIS2_PLACEMENT_3D('',#21542,#17579,#17580);
#15381=AXIS2_PLACEMENT_3D('',#21545,#17582,#17583);
#15382=AXIS2_PLACEMENT_3D('',#21546,#17584,#17585);
#15383=AXIS2_PLACEMENT_3D('',#21550,#17588,#17589);
#15384=AXIS2_PLACEMENT_3D('',#21552,#17591,#17592);
#15385=AXIS2_PLACEMENT_3D('',#21555,#17595,#17596);
#15386=AXIS2_PLACEMENT_3D('',#21557,#17598,#17599);
#15387=AXIS2_PLACEMENT_3D('',#21559,#17601,#17602);
#15388=AXIS2_PLACEMENT_3D('',#21561,#17604,#17605);
#15389=AXIS2_PLACEMENT_3D('',#21565,#17608,#17609);
#15390=AXIS2_PLACEMENT_3D('',#21568,#17611,#17612);
#15391=AXIS2_PLACEMENT_3D('',#21569,#17613,#17614);
#15392=AXIS2_PLACEMENT_3D('',#21573,#17617,#17618);
#15393=AXIS2_PLACEMENT_3D('',#21574,#17619,#17620);
#15394=AXIS2_PLACEMENT_3D('',#21575,#17621,#17622);
#15395=AXIS2_PLACEMENT_3D('',#21578,#17625,#17626);
#15396=AXIS2_PLACEMENT_3D('',#21580,#17628,#17629);
#15397=AXIS2_PLACEMENT_3D('',#21581,#17630,#17631);
#15398=AXIS2_PLACEMENT_3D('',#21582,#17632,#17633);
#15399=AXIS2_PLACEMENT_3D('',#21584,#17635,#17636);
#15400=AXIS2_PLACEMENT_3D('',#21586,#17638,#17639);
#15401=AXIS2_PLACEMENT_3D('',#21588,#17641,#17642);
#15402=AXIS2_PLACEMENT_3D('',#21590,#17644,#17645);
#17417=DIRECTION('axis',(0.,0.,1.));
#17418=DIRECTION('refdir',(1.,0.,0.));
#17419=DIRECTION('center_axis',(0.,-1.,0.));
#17420=DIRECTION('ref_axis',(1.,0.,0.));
#17421=DIRECTION('center_axis',(0.,-1.,0.));
#17422=DIRECTION('ref_axis',(1.,0.,0.));
#17423=DIRECTION('',(0.707106781186547,0.707106781186547,8.65956056235493E-17));
#17424=DIRECTION('center_axis',(0.,1.,0.));
#17425=DIRECTION('ref_axis',(1.,0.,0.));
#17426=DIRECTION('center_axis',(0.,-1.,0.));
#17427=DIRECTION('ref_axis',(1.,0.,0.));
#17428=DIRECTION('center_axis',(0.,-1.,0.));
#17429=DIRECTION('ref_axis',(1.,0.,0.));
#17430=DIRECTION('',(0.,-1.,0.));
#17431=DIRECTION('center_axis',(0.,1.,0.));
#17432=DIRECTION('ref_axis',(1.,0.,0.));
#17433=DIRECTION('',(-1.,0.,0.));
#17434=DIRECTION('center_axis',(0.,1.,0.));
#17435=DIRECTION('ref_axis',(0.707106781186547,0.,-0.707106781186547));
#17436=DIRECTION('',(0.,0.,-1.));
#17437=DIRECTION('center_axis',(0.,1.,0.));
#17438=DIRECTION('ref_axis',(0.707106781186547,0.,0.707106781186547));
#17439=DIRECTION('',(1.,0.,0.));
#17440=DIRECTION('center_axis',(0.,1.,0.));
#17441=DIRECTION('ref_axis',(-0.707106781186545,0.,0.70710678118655));
#17442=DIRECTION('',(0.,0.,1.));
#17443=DIRECTION('center_axis',(0.,1.,0.));
#17444=DIRECTION('ref_axis',(-0.707106781186547,0.,-0.707106781186547));
#17445=DIRECTION('center_axis',(0.,1.,0.));
#17446=DIRECTION('ref_axis',(1.,0.,0.));
#17447=DIRECTION('center_axis',(0.,1.,0.));
#17448=DIRECTION('ref_axis',(1.,0.,0.));
#17449=DIRECTION('center_axis',(0.,1.,0.));
#17450=DIRECTION('ref_axis',(1.,0.,0.));
#17451=DIRECTION('center_axis',(0.,1.,0.));
#17452=DIRECTION('ref_axis',(1.,0.,0.));
#17453=DIRECTION('',(0.707106781186547,-0.707106781186547,-8.65956056235493E-17));
#17454=DIRECTION('center_axis',(0.,1.,0.));
#17455=DIRECTION('ref_axis',(0.,0.,1.));
#17456=DIRECTION('',(-1.,0.,0.));
#17457=DIRECTION('center_axis',(0.,-1.,0.));
#17458=DIRECTION('ref_axis',(0.707106781186547,0.,0.707106781186547));
#17459=DIRECTION('',(0.,0.,1.));
#17460=DIRECTION('center_axis',(0.,-1.,0.));
#17461=DIRECTION('ref_axis',(0.707106781186547,0.,-0.707106781186547));
#17462=DIRECTION('',(1.,0.,0.));
#17463=DIRECTION('center_axis',(0.,-1.,0.));
#17464=DIRECTION('ref_axis',(-0.707106781186548,0.,-0.707106781186548));
#17465=DIRECTION('',(0.,0.,-1.));
#17466=DIRECTION('center_axis',(0.,-1.,0.));
#17467=DIRECTION('ref_axis',(-0.707106781186545,0.,0.70710678118655));
#17468=DIRECTION('center_axis',(0.,-1.,0.));
#17469=DIRECTION('ref_axis',(1.,0.,0.));
#17470=DIRECTION('center_axis',(0.,-1.,0.));
#17471=DIRECTION('ref_axis',(1.,0.,0.));
#17472=DIRECTION('center_axis',(0.,-0.70710678118654,-0.707106781186555));
#17473=DIRECTION('ref_axis',(-1.,0.,0.));
#17474=DIRECTION('',(0.,-0.707106781186555,0.70710678118654));
#17475=DIRECTION('',(0.,0.707106781186555,-0.70710678118654));
#17476=DIRECTION('',(1.,0.,0.));
#17477=DIRECTION('center_axis',(0.,1.,0.));
#17478=DIRECTION('ref_axis',(0.707106781186548,0.,-0.707106781186548));
#17479=DIRECTION('center_axis',(0.,-1.,0.));
#17480=DIRECTION('ref_axis',(0.707106781186548,0.,-0.707106781186548));
#17481=DIRECTION('',(-0.70710678118654,-0.707106781186555,0.));
#17482=DIRECTION('center_axis',(0.707106781186555,-0.70710678118654,0.));
#17483=DIRECTION('ref_axis',(0.,0.,-1.));
#17484=DIRECTION('',(-0.70710678118654,-0.707106781186555,0.));
#17485=DIRECTION('',(0.,0.,1.));
#17486=DIRECTION('center_axis',(0.,1.,0.));
#17487=DIRECTION('ref_axis',(0.707106781186548,0.,0.707106781186548));
#17488=DIRECTION('center_axis',(0.,-1.,0.));
#17489=DIRECTION('ref_axis',(0.707106781186548,0.,0.707106781186548));
#17490=DIRECTION('',(0.,-0.707106781186555,-0.70710678118654));
#17491=DIRECTION('center_axis',(0.,-0.70710678118654,0.707106781186555));
#17492=DIRECTION('ref_axis',(1.,0.,0.));
#17493=DIRECTION('',(0.,-0.707106781186555,-0.70710678118654));
#17494=DIRECTION('',(-1.,0.,0.));
#17495=DIRECTION('center_axis',(0.,1.,0.));
#17496=DIRECTION('ref_axis',(-0.707106781186545,0.,0.70710678118655));
#17497=DIRECTION('center_axis',(0.,-1.,0.));
#17498=DIRECTION('ref_axis',(-0.707106781186545,0.,0.70710678118655));
#17499=DIRECTION('',(0.707106781186524,-0.707106781186571,0.));
#17500=DIRECTION('center_axis',(-0.707106781186555,-0.70710678118654,0.));
#17501=DIRECTION('ref_axis',(0.,0.,1.));
#17502=DIRECTION('',(0.70710678118654,-0.707106781186555,0.));
#17503=DIRECTION('',(0.,0.,-1.));
#17504=DIRECTION('center_axis',(0.,1.,0.));
#17505=DIRECTION('ref_axis',(-0.707106781186548,0.,-0.707106781186548));
#17506=DIRECTION('center_axis',(0.,-1.,0.));
#17507=DIRECTION('ref_axis',(-0.707106781186548,0.,-0.707106781186548));
#17508=DIRECTION('center_axis',(0.,1.,0.));
#17509=DIRECTION('ref_axis',(0.707106781186548,0.,0.707106781186548));
#17510=DIRECTION('',(0.,1.,0.));
#17511=DIRECTION('center_axis',(0.,1.,0.));
#17512=DIRECTION('ref_axis',(0.707106781186548,0.,0.707106781186548));
#17513=DIRECTION('',(0.,-1.,0.));
#17514=DIRECTION('center_axis',(1.,0.,0.));
#17515=DIRECTION('ref_axis',(0.,0.,-1.));
#17516=DIRECTION('',(0.,-1.,0.));
#17517=DIRECTION('',(0.,0.,-1.));
#17518=DIRECTION('center_axis',(0.,1.,0.));
#17519=DIRECTION('ref_axis',(0.707106781186548,0.,-0.707106781186548));
#17520=DIRECTION('',(0.,1.,0.));
#17521=DIRECTION('center_axis',(0.,1.,0.));
#17522=DIRECTION('ref_axis',(0.707106781186548,0.,-0.707106781186548));
#17523=DIRECTION('center_axis',(0.,0.,-1.));
#17524=DIRECTION('ref_axis',(-1.,0.,0.));
#17525=DIRECTION('',(0.,-1.,0.));
#17526=DIRECTION('',(-1.,0.,0.));
#17527=DIRECTION('center_axis',(0.,0.382683432365099,0.923879532511283));
#17528=DIRECTION('ref_axis',(1.,0.,0.));
#17529=DIRECTION('',(0.,0.923879532511284,-0.382683432365096));
#17530=DIRECTION('',(-1.,0.,0.));
#17531=DIRECTION('',(0.,-0.923879532511284,0.382683432365096));
#17532=DIRECTION('',(1.,0.,0.));
#17533=DIRECTION('center_axis',(0.,-1.,0.));
#17534=DIRECTION('ref_axis',(0.707106781186548,0.,0.707106781186548));
#17535=DIRECTION('',(-0.382683432365087,0.923879532511288,0.));
#17536=DIRECTION('center_axis',(0.,-1.,0.));
#17537=DIRECTION('ref_axis',(0.707106781186548,0.,0.707106781186548));
#17538=DIRECTION('center_axis',(0.923879532511283,0.382683432365099,0.));
#17539=DIRECTION('ref_axis',(0.,0.,-1.));
#17540=DIRECTION('',(-0.382683432365096,0.923879532511284,0.));
#17541=DIRECTION('',(0.,0.,1.));
#17542=DIRECTION('center_axis',(0.,-1.,0.));
#17543=DIRECTION('ref_axis',(0.707106781186548,0.,-0.707106781186548));
#17544=DIRECTION('',(0.,0.923879532511288,0.382683432365087));
#17545=DIRECTION('center_axis',(0.,-1.,0.));
#17546=DIRECTION('ref_axis',(0.707106781186548,0.,-0.707106781186548));
#17547=DIRECTION('center_axis',(0.,0.382683432365099,-0.923879532511283));
#17548=DIRECTION('ref_axis',(-1.,0.,0.));
#17549=DIRECTION('',(0.,0.923879532511284,0.382683432365096));
#17550=DIRECTION('',(1.,0.,0.));
#17551=DIRECTION('center_axis',(0.,-1.,0.));
#17552=DIRECTION('ref_axis',(-0.707106781186549,0.,-0.707106781186546));
#17553=DIRECTION('',(0.382683432365086,0.923879532511288,0.));
#17554=DIRECTION('center_axis',(0.,-1.,0.));
#17555=DIRECTION('ref_axis',(-0.707106781186551,0.,-0.707106781186544));
#17556=DIRECTION('center_axis',(0.,1.,0.));
#17557=DIRECTION('ref_axis',(-0.707106781186548,0.,-0.707106781186548));
#17558=DIRECTION('center_axis',(-0.923879532511287,0.38268343236509,0.));
#17559=DIRECTION('ref_axis',(0.,0.,1.));
#17560=DIRECTION('',(0.38268343236509,0.923879532511286,0.));
#17561=DIRECTION('',(0.,0.,-1.));
#17562=DIRECTION('',(0.,0.,1.));
#17563=DIRECTION('center_axis',(0.,-1.,0.));
#17564=DIRECTION('ref_axis',(-0.707106781186544,0.,0.707106781186551));
#17565=DIRECTION('center_axis',(0.,-1.,0.));
#17566=DIRECTION('ref_axis',(-0.707106781186543,0.,0.707106781186552));
#17567=DIRECTION('center_axis',(0.,1.,0.));
#17568=DIRECTION('ref_axis',(-0.707106781186545,0.,0.70710678118655));
#17569=DIRECTION('center_axis',(0.,-1.,0.));
#17570=DIRECTION('ref_axis',(-0.707106781186547,0.,-0.707106781186547));
#17571=DIRECTION('',(-0.707106781186546,-0.707106781186549,0.));
#17572=DIRECTION('center_axis',(0.,1.,0.));
#17573=DIRECTION('ref_axis',(-0.707106781186551,0.,-0.707106781186544));
#17574=DIRECTION('',(0.,-0.707106781186543,-0.707106781186552));
#17575=DIRECTION('center_axis',(-0.707106781186549,0.707106781186546,0.));
#17576=DIRECTION('ref_axis',(0.,0.,1.));
#17577=DIRECTION('',(-0.70710678118654,-0.707106781186555,0.));
#17578=DIRECTION('',(0.,0.,1.));
#17579=DIRECTION('center_axis',(0.,-1.,0.));
#17580=DIRECTION('ref_axis',(-0.707106781186545,0.,0.70710678118655));
#17581=DIRECTION('',(0.,-0.707106781186549,0.707106781186546));
#17582=DIRECTION('center_axis',(0.,1.,0.));
#17583=DIRECTION('ref_axis',(-0.707106781186546,0.,0.707106781186549));
#17584=DIRECTION('center_axis',(0.,0.707106781186546,0.707106781186549));
#17585=DIRECTION('ref_axis',(1.,0.,0.));
#17586=DIRECTION('',(0.,-0.707106781186543,0.707106781186552));
#17587=DIRECTION('',(1.,0.,0.));
#17588=DIRECTION('center_axis',(0.,0.,1.));
#17589=DIRECTION('ref_axis',(1.,0.,0.));
#17590=DIRECTION('',(0.,1.,0.));
#17591=DIRECTION('center_axis',(0.,0.923879532511283,0.382683432365099));
#17592=DIRECTION('ref_axis',(0.,-0.382683432365099,0.923879532511283));
#17593=DIRECTION('',(0.,-0.382683432365094,0.923879532511285));
#17594=DIRECTION('',(0.,0.382683432365104,-0.923879532511281));
#17595=DIRECTION('center_axis',(0.,-1.,0.));
#17596=DIRECTION('ref_axis',(-0.707106781186546,0.,0.70710678118655));
#17597=DIRECTION('',(-0.923879532511281,-0.382683432365103,0.));
#17598=DIRECTION('center_axis',(-0.38268343236511,0.923879532511278,0.));
#17599=DIRECTION('ref_axis',(0.,0.,1.));
#17600=DIRECTION('',(-0.923879532511276,-0.382683432365115,0.));
#17601=DIRECTION('center_axis',(0.,-1.,0.));
#17602=DIRECTION('ref_axis',(-0.70710678118655,0.,-0.707106781186545));
#17603=DIRECTION('',(0.,-0.382683432365102,-0.923879532511282));
#17604=DIRECTION('center_axis',(0.,0.923879532511283,-0.382683432365099));
#17605=DIRECTION('ref_axis',(0.,0.382683432365099,0.923879532511283));
#17606=DIRECTION('',(0.,-0.382683432365094,-0.923879532511285));
#17607=DIRECTION('',(-1.,0.,0.));
#17608=DIRECTION('center_axis',(0.,-1.,0.));
#17609=DIRECTION('ref_axis',(0.707106781186548,0.,-0.707106781186548));
#17610=DIRECTION('',(0.923879532511287,-0.382683432365089,0.));
#17611=DIRECTION('center_axis',(0.,1.,0.));
#17612=DIRECTION('ref_axis',(0.707106781186547,0.,-0.707106781186547));
#17613=DIRECTION('center_axis',(0.382683432365109,0.923879532511279,0.));
#17614=DIRECTION('ref_axis',(0.,0.,1.));
#17615=DIRECTION('',(0.923879532511275,-0.382683432365119,0.));
#17616=DIRECTION('',(0.,0.,-1.));
#17617=DIRECTION('center_axis',(0.,-1.,0.));
#17618=DIRECTION('ref_axis',(0.707106781186548,0.,0.707106781186548));
#17619=DIRECTION('center_axis',(0.,1.,0.));
#17620=DIRECTION('ref_axis',(0.707106781186547,0.,0.707106781186547));
#17621=DIRECTION('center_axis',(0.,-1.,0.));
#17622=DIRECTION('ref_axis',(0.707106781186547,0.,-0.707106781186547));
#17623=DIRECTION('',(0.,-0.707106781186549,-0.707106781186546));
#17624=DIRECTION('',(0.707106781186552,-0.707106781186543,0.));
#17625=DIRECTION('center_axis',(0.707106781186549,0.707106781186546,0.));
#17626=DIRECTION('ref_axis',(0.,0.,-1.));
#17627=DIRECTION('',(-0.707106781186552,0.707106781186543,0.));
#17628=DIRECTION('center_axis',(0.,-1.,0.));
#17629=DIRECTION('ref_axis',(0.707106781186547,0.,0.707106781186547));
#17630=DIRECTION('center_axis',(0.,0.707106781186546,-0.707106781186549));
#17631=DIRECTION('ref_axis',(-1.,0.,0.));
#17632=DIRECTION('center_axis',(0.,-1.,0.));
#17633=DIRECTION('ref_axis',(1.,0.,0.));
#17634=DIRECTION('',(0.,-1.,0.));
#17635=DIRECTION('center_axis',(0.,-1.,0.));
#17636=DIRECTION('ref_axis',(1.,0.,0.));
#17637=DIRECTION('',(0.,-1.,0.));
#17638=DIRECTION('center_axis',(0.,1.,0.));
#17639=DIRECTION('ref_axis',(-0.707106781186548,0.,-0.707106781186548));
#17640=DIRECTION('',(0.,1.,0.));
#17641=DIRECTION('center_axis',(0.,1.,0.));
#17642=DIRECTION('ref_axis',(-0.707106781186545,0.,0.70710678118655));
#17643=DIRECTION('',(0.,-1.,0.));
#17644=DIRECTION('center_axis',(-1.,0.,0.));
#17645=DIRECTION('ref_axis',(0.,0.,1.));
#21386=CARTESIAN_POINT('',(0.,0.,0.));
#21387=CARTESIAN_POINT('Origin',(24.,8.1,-47.5));
#21388=CARTESIAN_POINT('',(19.6,8.,-47.5));
#21389=CARTESIAN_POINT('Origin',(24.,8.,-47.5));
#21390=CARTESIAN_POINT('',(19.8,8.2,-47.5));
#21391=CARTESIAN_POINT('',(19.7,8.1,-47.5));
#21392=CARTESIAN_POINT('Origin',(24.,8.2,-47.5));
#21393=CARTESIAN_POINT('Origin',(24.,11.,-47.5));
#21394=CARTESIAN_POINT('',(19.8,10.8,-47.5));
#21395=CARTESIAN_POINT('Origin',(24.,10.8,-47.5));
#21396=CARTESIAN_POINT('',(19.8,11.,-47.5));
#21397=CARTESIAN_POINT('Origin',(3.99999999999999,8.,-47.5));
#21398=CARTESIAN_POINT('',(43.5,8.,-54.8));
#21399=CARTESIAN_POINT('',(-35.5,8.,-54.8));
#21400=CARTESIAN_POINT('',(24.5,8.,-54.8));
#21401=CARTESIAN_POINT('',(44.8,8.,-53.5));
#21402=CARTESIAN_POINT('Origin',(43.5,8.,-53.5));
#21403=CARTESIAN_POINT('',(44.8,8.,-41.5));
#21404=CARTESIAN_POINT('',(44.8,8.,-43.75));
#21405=CARTESIAN_POINT('',(43.5,8.,-40.2));
#21406=CARTESIAN_POINT('Origin',(43.5,8.,-41.5));
#21407=CARTESIAN_POINT('',(-35.5,8.,-40.2));
#21408=CARTESIAN_POINT('',(-16.5,8.,-40.2));
#21409=CARTESIAN_POINT('',(-36.8,8.,-41.5));
#21410=CARTESIAN_POINT('Origin',(-35.5,8.,-41.5));
#21411=CARTESIAN_POINT('',(-36.8,8.,-53.5));
#21412=CARTESIAN_POINT('',(-36.8,8.,-51.25));
#21413=CARTESIAN_POINT('Origin',(-35.5,8.,-53.5));
#21414=CARTESIAN_POINT('',(-35.7,8.,-47.5));
#21415=CARTESIAN_POINT('Origin',(-34.25,8.,-47.5));
#21416=CARTESIAN_POINT('',(40.8,8.,-47.5));
#21417=CARTESIAN_POINT('Origin',(42.25,8.,-47.5));
#21418=CARTESIAN_POINT('Origin',(24.,10.9,-47.5));
#21419=CARTESIAN_POINT('',(19.6,11.,-47.5));
#21420=CARTESIAN_POINT('Origin',(24.,11.,-47.5));
#21421=CARTESIAN_POINT('',(19.7,10.9,-47.5));
#21422=CARTESIAN_POINT('Origin',(3.99999999999999,11.,-47.5));
#21423=CARTESIAN_POINT('',(43.5,11.,-40.7));
#21424=CARTESIAN_POINT('',(-35.5,11.,-40.7));
#21425=CARTESIAN_POINT('',(-6.25,11.,-40.7));
#21426=CARTESIAN_POINT('',(44.3,11.,-41.5));
#21427=CARTESIAN_POINT('Origin',(43.5,11.,-41.5));
#21428=CARTESIAN_POINT('',(44.3,11.,-53.5));
#21429=CARTESIAN_POINT('',(44.3,11.,-45.625));
#21430=CARTESIAN_POINT('',(43.5,11.,-54.3));
#21431=CARTESIAN_POINT('Origin',(43.5,11.,-53.5));
#21432=CARTESIAN_POINT('',(-35.5,11.,-54.3));
#21433=CARTESIAN_POINT('',(14.25,11.,-54.3));
#21434=CARTESIAN_POINT('',(-36.3,11.,-53.5));
#21435=CARTESIAN_POINT('Origin',(-35.5,11.,-53.5));
#21436=CARTESIAN_POINT('',(-36.3,11.,-41.5));
#21437=CARTESIAN_POINT('',(-36.3,11.,-49.375));
#21438=CARTESIAN_POINT('Origin',(-35.5,11.,-41.5));
#21439=CARTESIAN_POINT('',(40.8,11.,-47.5));
#21440=CARTESIAN_POINT('Origin',(42.25,11.,-47.5));
#21441=CARTESIAN_POINT('',(-35.7,11.,-47.5));
#21442=CARTESIAN_POINT('Origin',(-34.25,11.,-47.5));
#21443=CARTESIAN_POINT('Origin',(24.5,8.1,-54.9));
#21444=CARTESIAN_POINT('',(43.5,8.2,-55.));
#21445=CARTESIAN_POINT('',(43.5,8.2,-55.));
#21446=CARTESIAN_POINT('',(-35.5,8.2,-55.));
#21447=CARTESIAN_POINT('',(-35.5,8.,-54.8));
#21448=CARTESIAN_POINT('',(24.5,8.2,-55.));
#21449=CARTESIAN_POINT('Origin',(43.5,8.1,-53.5));
#21450=CARTESIAN_POINT('',(45.,8.2,-53.5));
#21451=CARTESIAN_POINT('Origin',(43.5,8.2,-53.5));
#21452=CARTESIAN_POINT('',(45.,8.2,-53.5));
#21453=CARTESIAN_POINT('Origin',(44.9,8.1,-43.75));
#21454=CARTESIAN_POINT('',(45.,8.2,-41.5));
#21455=CARTESIAN_POINT('',(45.,8.2,-41.5));
#21456=CARTESIAN_POINT('',(45.,8.2,-43.75));
#21457=CARTESIAN_POINT('Origin',(43.5,8.1,-41.5));
#21458=CARTESIAN_POINT('',(43.5,8.2,-40.));
#21459=CARTESIAN_POINT('Origin',(43.5,8.2,-41.5));
#21460=CARTESIAN_POINT('',(43.5,8.2,-40.));
#21461=CARTESIAN_POINT('Origin',(-16.5,8.1,-40.1));
#21462=CARTESIAN_POINT('',(-35.5,8.2,-40.));
#21463=CARTESIAN_POINT('',(-35.5,8.2,-40.));
#21464=CARTESIAN_POINT('',(-16.5,8.2,-40.));
#21465=CARTESIAN_POINT('Origin',(-35.5,8.1,-41.5));
#21466=CARTESIAN_POINT('',(-37.,8.2,-41.5));
#21467=CARTESIAN_POINT('Origin',(-35.5,8.2,-41.5));
#21468=CARTESIAN_POINT('',(-37.,8.2,-41.5));
#21469=CARTESIAN_POINT('Origin',(-36.9,8.1,-51.25));
#21470=CARTESIAN_POINT('',(-37.,8.2,-53.5));
#21471=CARTESIAN_POINT('',(-37.,8.2,-53.5));
#21472=CARTESIAN_POINT('',(-37.,8.2,-51.25));
#21473=CARTESIAN_POINT('Origin',(-35.5,8.1,-53.5));
#21474=CARTESIAN_POINT('Origin',(-35.5,8.2,-53.5));
#21475=CARTESIAN_POINT('Origin',(43.5,8.,-41.5));
#21476=CARTESIAN_POINT('',(45.,10.3,-41.5));
#21477=CARTESIAN_POINT('',(45.,8.,-41.5));
#21478=CARTESIAN_POINT('',(43.5,10.3,-40.));
#21479=CARTESIAN_POINT('Origin',(43.5,10.3,-41.5));
#21480=CARTESIAN_POINT('',(43.5,8.,-40.));
#21481=CARTESIAN_POINT('Origin',(45.,8.,-40.));
#21482=CARTESIAN_POINT('',(45.,10.3,-53.5));
#21483=CARTESIAN_POINT('',(45.,8.,-53.5));
#21484=CARTESIAN_POINT('',(45.,10.3,-41.875));
#21485=CARTESIAN_POINT('Origin',(43.5,8.,-53.5));
#21486=CARTESIAN_POINT('',(43.5,10.3,-55.));
#21487=CARTESIAN_POINT('',(43.5,8.,-55.));
#21488=CARTESIAN_POINT('Origin',(43.5,10.3,-53.5));
#21489=CARTESIAN_POINT('Origin',(45.,8.,-55.));
#21490=CARTESIAN_POINT('',(-35.5,10.3,-55.));
#21491=CARTESIAN_POINT('',(-35.5,8.,-55.));
#21492=CARTESIAN_POINT('',(34.75,10.3,-55.));
#21493=CARTESIAN_POINT('Origin',(-26.75,10.4707106781187,-40.0707106781187));
#21494=CARTESIAN_POINT('',(43.5,10.6414213562373,-40.1414213562373));
#21495=CARTESIAN_POINT('',(43.5,10.3,-40.));
#21496=CARTESIAN_POINT('',(-35.5,10.6414213562373,-40.1414213562373));
#21497=CARTESIAN_POINT('',(-26.75,10.6414213562373,-40.1414213562373));
#21498=CARTESIAN_POINT('',(-35.5,10.3,-40.));
#21499=CARTESIAN_POINT('',(-35.5,10.6414213562373,-40.1414213562373));
#21500=CARTESIAN_POINT('',(-26.75,10.3,-40.));
#21501=CARTESIAN_POINT('Origin',(43.5,10.4707106781187,-41.5));
#21502=CARTESIAN_POINT('',(44.8585786437627,10.6414213562373,-41.5));
#21503=CARTESIAN_POINT('',(45.,10.3,-41.5));
#21504=CARTESIAN_POINT('Origin',(43.5,10.6414213562373,-41.5));
#21505=CARTESIAN_POINT('Origin',(44.9292893218813,10.4707106781187,-41.875));
#21506=CARTESIAN_POINT('',(44.8585786437627,10.6414213562373,-53.5));
#21507=CARTESIAN_POINT('',(45.,10.3,-53.5));
#21508=CARTESIAN_POINT('',(44.8585786437627,10.6414213562373,-41.875));
#21509=CARTESIAN_POINT('Origin',(43.5,10.4707106781187,-53.5));
#21510=CARTESIAN_POINT('',(43.5,10.6414213562373,-54.8585786437627));
#21511=CARTESIAN_POINT('',(43.5,10.3,-55.));
#21512=CARTESIAN_POINT('Origin',(43.5,10.6414213562373,-53.5));
#21513=CARTESIAN_POINT('Origin',(34.75,10.4707106781187,-54.9292893218813));
#21514=CARTESIAN_POINT('',(-35.5,10.6414213562373,-54.8585786437627));
#21515=CARTESIAN_POINT('',(-35.5,10.3,-55.));
#21516=CARTESIAN_POINT('',(34.75,10.6414213562373,-54.8585786437627));
#21517=CARTESIAN_POINT('Origin',(-35.5,10.4707106781187,-53.5));
#21518=CARTESIAN_POINT('',(-37.,10.3,-53.5));
#21519=CARTESIAN_POINT('',(-36.8585786437627,10.6414213562373,-53.5));
#21520=CARTESIAN_POINT('',(-37.,10.3,-53.5));
#21521=CARTESIAN_POINT('Origin',(-35.5,10.6414213562373,-53.5));
#21522=CARTESIAN_POINT('Origin',(-35.5,10.3,-53.5));
#21523=CARTESIAN_POINT('Origin',(-36.9292893218813,10.4707106781187,-53.125));
#21524=CARTESIAN_POINT('',(-37.,10.3,-41.5));
#21525=CARTESIAN_POINT('',(-36.8585786437627,10.6414213562373,-41.5));
#21526=CARTESIAN_POINT('',(-37.,10.3,-41.5));
#21527=CARTESIAN_POINT('',(-36.8585786437627,10.6414213562373,-53.125));
#21528=CARTESIAN_POINT('',(-37.,10.3,-53.125));
#21529=CARTESIAN_POINT('Origin',(-35.5,10.4707106781187,-41.5));
#21530=CARTESIAN_POINT('Origin',(-35.5,10.6414213562373,-41.5));
#21531=CARTESIAN_POINT('Origin',(-35.5,10.3,-41.5));
#21532=CARTESIAN_POINT('Origin',(-35.5,10.75,-53.5));
#21533=CARTESIAN_POINT('',(-36.6414213562373,10.8585786437627,-53.5));
#21534=CARTESIAN_POINT('',(-36.5,11.,-53.5));
#21535=CARTESIAN_POINT('',(-35.5,10.8585786437627,-54.6414213562373));
#21536=CARTESIAN_POINT('Origin',(-35.5,10.8585786437627,-53.5));
#21537=CARTESIAN_POINT('',(-35.5,11.,-54.5));
#21538=CARTESIAN_POINT('Origin',(-36.75,10.75,-51.25));
#21539=CARTESIAN_POINT('',(-36.6414213562373,10.8585786437627,-41.5));
#21540=CARTESIAN_POINT('',(-36.5,11.,-41.5));
#21541=CARTESIAN_POINT('',(-36.6414213562373,10.8585786437627,-49.375));
#21542=CARTESIAN_POINT('Origin',(-35.5,10.75,-41.5));
#21543=CARTESIAN_POINT('',(-35.5,10.8585786437627,-40.3585786437627));
#21544=CARTESIAN_POINT('',(-35.5,11.,-40.5));
#21545=CARTESIAN_POINT('Origin',(-35.5,10.8585786437627,-41.5));
#21546=CARTESIAN_POINT('Origin',(-16.5,10.75,-40.25));
#21547=CARTESIAN_POINT('',(43.5,10.8585786437627,-40.3585786437627));
#21548=CARTESIAN_POINT('',(43.5,11.,-40.5));
#21549=CARTESIAN_POINT('',(-6.25,10.8585786437627,-40.3585786437627));
#21550=CARTESIAN_POINT('Origin',(-37.,8.,-40.));
#21551=CARTESIAN_POINT('',(-35.5,8.,-40.));
#21552=CARTESIAN_POINT('Origin',(-6.25,10.9292893218813,-40.5292893218813));
#21553=CARTESIAN_POINT('',(-35.5,11.,-40.7));
#21554=CARTESIAN_POINT('',(43.5,10.8585786437627,-40.3585786437627));
#21555=CARTESIAN_POINT('Origin',(-35.5,10.9292893218813,-41.5));
#21556=CARTESIAN_POINT('',(-36.3,11.,-41.5));
#21557=CARTESIAN_POINT('Origin',(-36.4707106781187,10.9292893218813,-49.375));
#21558=CARTESIAN_POINT('',(-36.3,11.,-53.5));
#21559=CARTESIAN_POINT('Origin',(-35.5,10.9292893218813,-53.5));
#21560=CARTESIAN_POINT('',(-35.5,11.,-54.3));
#21561=CARTESIAN_POINT('Origin',(14.25,10.9292893218813,-54.4707106781187));
#21562=CARTESIAN_POINT('',(43.5,10.8585786437627,-54.6414213562373));
#21563=CARTESIAN_POINT('',(43.5,11.,-54.3));
#21564=CARTESIAN_POINT('',(14.25,10.8585786437627,-54.6414213562373));
#21565=CARTESIAN_POINT('Origin',(43.5,10.9292893218813,-53.5));
#21566=CARTESIAN_POINT('',(44.6414213562373,10.8585786437627,-53.5));
#21567=CARTESIAN_POINT('',(44.3,11.,-53.5));
#21568=CARTESIAN_POINT('Origin',(43.5,10.8585786437627,-53.5));
#21569=CARTESIAN_POINT('Origin',(44.4707106781187,10.9292893218813,-45.625));
#21570=CARTESIAN_POINT('',(44.6414213562373,10.8585786437627,-41.5));
#21571=CARTESIAN_POINT('',(44.3,11.,-41.5));
#21572=CARTESIAN_POINT('',(44.6414213562373,10.8585786437627,-45.625));
#21573=CARTESIAN_POINT('Origin',(43.5,10.9292893218813,-41.5));
#21574=CARTESIAN_POINT('Origin',(43.5,10.8585786437627,-41.5));
#21575=CARTESIAN_POINT('Origin',(43.5,10.75,-53.5));
#21576=CARTESIAN_POINT('',(43.5,11.,-54.5));
#21577=CARTESIAN_POINT('',(44.5,11.,-53.5));
#21578=CARTESIAN_POINT('Origin',(44.75,10.75,-43.75));
#21579=CARTESIAN_POINT('',(45.,10.5,-41.5));
#21580=CARTESIAN_POINT('Origin',(43.5,10.75,-41.5));
#21581=CARTESIAN_POINT('Origin',(24.5,10.75,-54.75));
#21582=CARTESIAN_POINT('Origin',(-34.25,11.,-47.5));
#21583=CARTESIAN_POINT('',(-35.7,11.,-47.5));
#21584=CARTESIAN_POINT('Origin',(42.25,11.,-47.5));
#21585=CARTESIAN_POINT('',(40.8,11.,-47.5));
#21586=CARTESIAN_POINT('Origin',(-35.5,8.,-53.5));
#21587=CARTESIAN_POINT('',(-37.,8.,-53.5));
#21588=CARTESIAN_POINT('Origin',(-35.5,8.,-41.5));
#21589=CARTESIAN_POINT('',(-37.,8.,-41.5));
#21590=CARTESIAN_POINT('Origin',(-37.,8.,-55.));
#37156=UNCERTAINTY_MEASURE_WITH_UNIT(LENGTH_MEASURE(0.01),#37182,
'DISTANCE_ACCURACY_VALUE',
'Maximum model space distance between geometric entities at asserted c
onnectivities');
#37166=UNCERTAINTY_MEASURE_WITH_UNIT(LENGTH_MEASURE(0.01),#37182,
'DISTANCE_ACCURACY_VALUE',
'Maximum model space distance between geometric entities at asserted c
onnectivities');
#37171=(
GEOMETRIC_REPRESENTATION_CONTEXT(3)
GLOBAL_UNCERTAINTY_ASSIGNED_CONTEXT((#37156))
GLOBAL_UNIT_ASSIGNED_CONTEXT((#37182,#37184,#37185))
REPRESENTATION_CONTEXT('','3D')
);
#37181=(
GEOMETRIC_REPRESENTATION_CONTEXT(3)
GLOBAL_UNCERTAINTY_ASSIGNED_CONTEXT((#37166))
GLOBAL_UNIT_ASSIGNED_CONTEXT((#37182,#37184,#37185))
REPRESENTATION_CONTEXT('','3D')
);
#37182=(
LENGTH_UNIT()
NAMED_UNIT(*)
SI_UNIT(.MILLI.,.METRE.)
);
#37184=(
NAMED_UNIT(*)
PLANE_ANGLE_UNIT()
SI_UNIT($,.RADIAN.)
);
#37185=(
NAMED_UNIT(*)
SI_UNIT($,.STERADIAN.)
SOLID_ANGLE_UNIT()
);
#37190=SHAPE_DEFINITION_REPRESENTATION(#37204,#37241);
#37204=PRODUCT_DEFINITION_SHAPE('',$,#37256);
#37241=SHAPE_REPRESENTATION('',(#15323),#37171);
#37251=PRODUCT_DEFINITION_CONTEXT('part definition',#37295,'design');
#37256=PRODUCT_DEFINITION('2026-10-20-13-23-53-005',
'04_Camera_Housing_Front_Cover_PLA',#37270,#37251);
#37270=PRODUCT_DEFINITION_FORMATION('',$,#37301);
#37295=APPLICATION_CONTEXT(
'Core Data for Automotive Mechanical Design Process');
#37296=PRODUCT_CONTEXT('part definition',#37295,'mechanical');
#37301=PRODUCT('2026-10-20-13-23-53-005',
'04_Camera_Housing_Front_Cover_PLA',$,(#37296));
#37346=COLOUR_RGB('Dark Blue',0.08,0.2,0.34);
#37347=FILL_AREA_STYLE_COLOUR('',#37346);
#37348=FILL_AREA_STYLE('',(#37347));
#37349=SURFACE_STYLE_FILL_AREA(#37348);
#37350=SURFACE_SIDE_STYLE('',(#37349));
#37351=SURFACE_STYLE_USAGE(.BOTH.,#37350);
#37352=PRESENTATION_STYLE_ASSIGNMENT((#37351));
ENDSEC;
END-ISO-10303-21;
